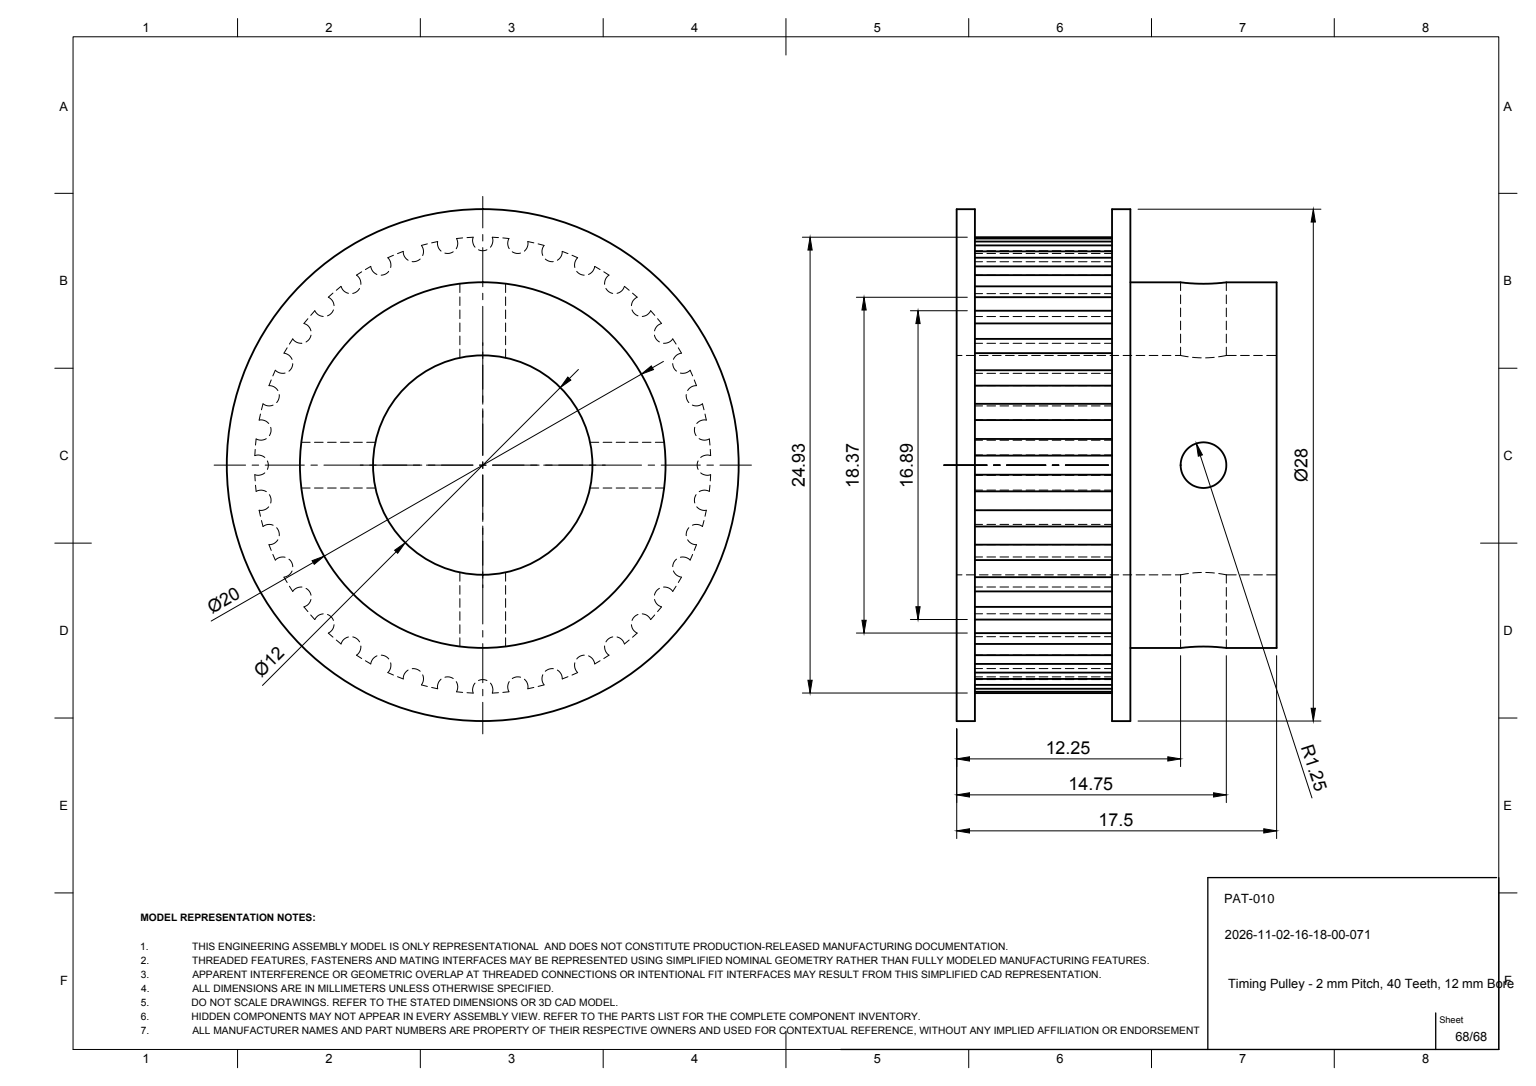
ISO-10303-21;
HEADER;
/* Generated by software containing ST-Developer
 * from STEP Tools, Inc. (www.steptools.com) 
 */

FILE_DESCRIPTION(
/* description */ ('Belt conveyor head drive unit'),
/* implementation_level */ '2;1');

FILE_NAME(
/* name */ 'Timing Pulley - 2 mm Pitch, 40 Teeth, 12 mm Bore.step',
/* time_stamp */ '2026-10-28T03:26:19-07:00',
/* author */ (''),
/* organization */ (''),
/* preprocessor_version */ 'ST-DEVELOPER v20.2',
/* originating_system */ 'Autodesk Translation Framework v15.17.0.0',
/* authorisation */ '');

FILE_SCHEMA (('AUTOMOTIVE_DESIGN { 1 0 10303 214 3 1 1 }'));
ENDSEC;

DATA;
#10=MECHANICAL_DESIGN_GEOMETRIC_PRESENTATION_REPRESENTATION('',(#929),#27069);
#623=B_SPLINE_CURVE_WITH_KNOTS('',3,(#25841,#25842,#25843,#25844,#25845,
#25846,#25847,#25848,#25849,#25850),.UNSPECIFIED.,.F.,.F.,(4,2,2,2,4),(0.565665723963061,
0.61280433739166,0.659942950820258,0.70708195805217,0.754220965284082),
 .UNSPECIFIED.);
#624=B_SPLINE_CURVE_WITH_KNOTS('',3,(#25852,#25853,#25854,#25855,#25856,
#25857,#25858,#25859,#25860,#25861,#25862,#25863,#25864,#25865,#25866,#25867,
#25868,#25869),.UNSPECIFIED.,.F.,.F.,(4,2,2,2,2,2,2,2,4),(0.18855524132102,
0.235693854749619,0.282832468178217,0.329971475410129,0.377110482642041,
0.424249489873953,0.471388497105864,0.518527110534463,0.565665723963061),
 .UNSPECIFIED.);
#625=B_SPLINE_CURVE_WITH_KNOTS('',3,(#25870,#25871,#25872,#25873,#25874,
#25875,#25876,#25877,#25878,#25879),.UNSPECIFIED.,.F.,.F.,(4,2,2,2,4),(0.754220965284082,
0.801359972515993,0.848498979747905,0.895637593176504,0.942776206605102),
 .UNSPECIFIED.);
#626=B_SPLINE_CURVE_WITH_KNOTS('',3,(#25883,#25884,#25885,#25886,#25887,
#25888,#25889,#25890,#25891,#25892),.UNSPECIFIED.,.F.,.F.,(4,2,2,2,4),(0.188940047579712,
0.236173496177583,0.283406944775455,0.330643519967439,0.377880095159423),
 .UNSPECIFIED.);
#627=B_SPLINE_CURVE_WITH_KNOTS('',3,(#25894,#25895,#25896,#25897,#25898,
#25899,#25900,#25901,#25902,#25903),.UNSPECIFIED.,.F.,.F.,(4,2,2,2,4),(0.,
0.0472365751919841,0.0944731503839682,0.14170659898184,0.188940047579712),
 .UNSPECIFIED.);
#628=B_SPLINE_CURVE_WITH_KNOTS('',3,(#25905,#25906,#25907,#25908,#25909,
#25910,#25911,#25912,#25913,#25914),.UNSPECIFIED.,.F.,.F.,(4,2,2,2,4),(0.566820142739135,
0.614053591337007,0.661287039934879,0.708523615126863,0.755760190318847),
 .UNSPECIFIED.);
#629=B_SPLINE_CURVE_WITH_KNOTS('',3,(#25915,#25916,#25917,#25918,#25919,
#25920,#25921,#25922,#25923,#25924),.UNSPECIFIED.,.F.,.F.,(4,2,2,2,4),(0.377880095159423,
0.425116670351408,0.472353245543392,0.519586694141263,0.566820142739135),
 .UNSPECIFIED.);
#630=B_SPLINE_CURVE_WITH_KNOTS('',3,(#25928,#25929,#25930,#25931,#25932,
#25933,#25934,#25935,#25936,#25937,#25938,#25939,#25940,#25941,#25942,#25943,
#25944,#25945),.UNSPECIFIED.,.F.,.F.,(4,2,2,2,2,2,2,2,4),(0.,0.0472365751919841,
0.0944731503839683,0.14170659898184,0.188940047579712,0.236173496177583,
0.283406944775455,0.330643519967439,0.377880095159423),.UNSPECIFIED.);
#631=B_SPLINE_CURVE_WITH_KNOTS('',3,(#25946,#25947,#25948,#25949,#25950,
#25951,#25952,#25953,#25954,#25955,#25956,#25957,#25958,#25959,#25960,#25961,
#25962,#25963),.UNSPECIFIED.,.F.,.F.,(4,2,2,2,2,2,2,2,4),(0.377880095159423,
0.425116670351408,0.472353245543392,0.519586694141263,0.566820142739135,
0.614053591337007,0.661287039934879,0.708523615126863,0.755760190318847),
 .UNSPECIFIED.);
#632=B_SPLINE_CURVE_WITH_KNOTS('',3,(#25967,#25968,#25969,#25970,#25971,
#25972,#25973,#25974,#25975,#25976),.UNSPECIFIED.,.F.,.F.,(4,2,2,2,4),(0.565665723963061,
0.61280433739166,0.659942950820258,0.70708195805217,0.754220965284082),
 .UNSPECIFIED.);
#633=B_SPLINE_CURVE_WITH_KNOTS('',3,(#25978,#25979,#25980,#25981,#25982,
#25983,#25984,#25985,#25986,#25987,#25988,#25989,#25990,#25991,#25992,#25993,
#25994,#25995),.UNSPECIFIED.,.F.,.F.,(4,2,2,2,2,2,2,2,4),(0.18855524132102,
0.235693854749619,0.282832468178217,0.329971475410129,0.377110482642041,
0.424249489873953,0.471388497105864,0.518527110534463,0.565665723963061),
 .UNSPECIFIED.);
#634=B_SPLINE_CURVE_WITH_KNOTS('',3,(#25996,#25997,#25998,#25999,#26000,
#26001,#26002,#26003,#26004,#26005),.UNSPECIFIED.,.F.,.F.,(4,2,2,2,4),(0.754220965284082,
0.801359972515993,0.848498979747905,0.895637593176504,0.942776206605102),
 .UNSPECIFIED.);
#635=B_SPLINE_CURVE_WITH_KNOTS('',3,(#26015,#26016,#26017,#26018,#26019,
#26020,#26021,#26022,#26023,#26024,#26025,#26026,#26027,#26028,#26029,#26030,
#26031,#26032),.UNSPECIFIED.,.F.,.F.,(4,2,2,2,2,2,2,2,4),(0.18855524132102,
0.235693854749619,0.282832468178217,0.329971475410129,0.377110482642041,
0.424249489873953,0.471388497105864,0.518527110534463,0.565665723963061),
 .UNSPECIFIED.);
#636=B_SPLINE_CURVE_WITH_KNOTS('',3,(#26034,#26035,#26036,#26037,#26038,
#26039,#26040,#26041,#26042,#26043),.UNSPECIFIED.,.F.,.F.,(4,2,2,2,4),(0.565665723963061,
0.61280433739166,0.659942950820258,0.70708195805217,0.754220965284082),
 .UNSPECIFIED.);
#637=B_SPLINE_CURVE_WITH_KNOTS('',3,(#26044,#26045,#26046,#26047,#26048,
#26049,#26050,#26051,#26052,#26053),.UNSPECIFIED.,.F.,.F.,(4,2,2,2,4),(0.754220965284082,
0.801359972515993,0.848498979747905,0.895637593176504,0.942776206605102),
 .UNSPECIFIED.);
#638=B_SPLINE_CURVE_WITH_KNOTS('',3,(#26056,#26057,#26058,#26059,#26060,
#26061,#26062,#26063,#26064,#26065,#26066,#26067,#26068,#26069,#26070,#26071,
#26072,#26073),.UNSPECIFIED.,.F.,.F.,(4,2,2,2,2,2,2,2,4),(0.18855524132102,
0.235693854749619,0.282832468178217,0.329971475410129,0.377110482642041,
0.424249489873953,0.471388497105864,0.518527110534463,0.565665723963061),
 .UNSPECIFIED.);
#639=B_SPLINE_CURVE_WITH_KNOTS('',3,(#26075,#26076,#26077,#26078,#26079,
#26080,#26081,#26082,#26083,#26084),.UNSPECIFIED.,.F.,.F.,(4,2,2,2,4),(0.565665723963061,
0.61280433739166,0.659942950820258,0.70708195805217,0.754220965284082),
 .UNSPECIFIED.);
#640=B_SPLINE_CURVE_WITH_KNOTS('',3,(#26085,#26086,#26087,#26088,#26089,
#26090,#26091,#26092,#26093,#26094),.UNSPECIFIED.,.F.,.F.,(4,2,2,2,4),(0.754220965284082,
0.801359972515993,0.848498979747905,0.895637593176504,0.942776206605102),
 .UNSPECIFIED.);
#641=B_SPLINE_CURVE_WITH_KNOTS('',3,(#26099,#26100,#26101,#26102,#26103,
#26104,#26105,#26106,#26107,#26108,#26109,#26110,#26111,#26112,#26113,#26114,
#26115,#26116),.UNSPECIFIED.,.F.,.F.,(4,2,2,2,2,2,2,2,4),(0.,0.0472365751919841,
0.0944731503839683,0.14170659898184,0.188940047579712,0.236173496177583,
0.283406944775455,0.330643519967439,0.377880095159424),.UNSPECIFIED.);
#642=B_SPLINE_CURVE_WITH_KNOTS('',3,(#26117,#26118,#26119,#26120,#26121,
#26122,#26123,#26124,#26125,#26126,#26127,#26128,#26129,#26130,#26131,#26132,
#26133,#26134),.UNSPECIFIED.,.F.,.F.,(4,2,2,2,2,2,2,2,4),(0.377880095159424,
0.425116670351408,0.472353245543392,0.519586694141263,0.566820142739135,
0.614053591337007,0.661287039934879,0.708523615126863,0.755760190318847),
 .UNSPECIFIED.);
#643=B_SPLINE_CURVE_WITH_KNOTS('',3,(#26138,#26139,#26140,#26141,#26142,
#26143,#26144,#26145,#26146,#26147,#26148,#26149,#26150,#26151,#26152,#26153,
#26154,#26155),.UNSPECIFIED.,.F.,.F.,(4,2,2,2,2,2,2,2,4),(0.,0.0472365751919841,
0.0944731503839683,0.14170659898184,0.188940047579712,0.236173496177583,
0.283406944775455,0.330643519967439,0.377880095159423),.UNSPECIFIED.);
#644=B_SPLINE_CURVE_WITH_KNOTS('',3,(#26156,#26157,#26158,#26159,#26160,
#26161,#26162,#26163,#26164,#26165,#26166,#26167,#26168,#26169,#26170,#26171,
#26172,#26173),.UNSPECIFIED.,.F.,.F.,(4,2,2,2,2,2,2,2,4),(0.377880095159423,
0.425116670351408,0.472353245543392,0.519586694141263,0.566820142739135,
0.614053591337007,0.661287039934879,0.708523615126863,0.755760190318847),
 .UNSPECIFIED.);
#775=SHAPE_REPRESENTATION_RELATIONSHIP('SRR','None',#27424,#844);
#844=ADVANCED_BREP_SHAPE_REPRESENTATION('',(#1010),#27066);
#929=STYLED_ITEM('',(#27790),#1010);
#1010=MANIFOLD_SOLID_BREP('Body1',#13798);
#1264=FACE_BOUND('',#3366,.T.);
#1265=FACE_BOUND('',#3367,.T.);
#1266=FACE_BOUND('',#3368,.T.);
#1267=FACE_BOUND('',#3372,.T.);
#1268=FACE_BOUND('',#3373,.T.);
#1269=FACE_BOUND('',#3374,.T.);
#1270=FACE_BOUND('',#3376,.T.);
#1271=FACE_BOUND('',#3378,.T.);
#1272=FACE_BOUND('',#3381,.T.);
#1273=FACE_BOUND('',#3383,.T.);
#1274=FACE_BOUND('',#3386,.T.);
#1608=PLANE('',#16027);
#1609=PLANE('',#16028);
#1610=PLANE('',#16112);
#1611=PLANE('',#16113);
#1612=PLANE('',#16197);
#2311=FACE_OUTER_BOUND('',#3363,.T.);
#2312=FACE_OUTER_BOUND('',#3364,.T.);
#2313=FACE_OUTER_BOUND('',#3365,.T.);
#2314=FACE_OUTER_BOUND('',#3369,.T.);
#2315=FACE_OUTER_BOUND('',#3370,.T.);
#2316=FACE_OUTER_BOUND('',#3371,.T.);
#2317=FACE_OUTER_BOUND('',#3375,.T.);
#2318=FACE_OUTER_BOUND('',#3377,.T.);
#2319=FACE_OUTER_BOUND('',#3379,.T.);
#2320=FACE_OUTER_BOUND('',#3380,.T.);
#2321=FACE_OUTER_BOUND('',#3382,.T.);
#2322=FACE_OUTER_BOUND('',#3384,.T.);
#2323=FACE_OUTER_BOUND('',#3385,.T.);
#2324=FACE_OUTER_BOUND('',#3387,.T.);
#2325=FACE_OUTER_BOUND('',#3388,.T.);
#2326=FACE_OUTER_BOUND('',#3389,.T.);
#2327=FACE_OUTER_BOUND('',#3390,.T.);
#2328=FACE_OUTER_BOUND('',#3391,.T.);
#2329=FACE_OUTER_BOUND('',#3392,.T.);
#2330=FACE_OUTER_BOUND('',#3393,.T.);
#2331=FACE_OUTER_BOUND('',#3394,.T.);
#2332=FACE_OUTER_BOUND('',#3395,.T.);
#2333=FACE_OUTER_BOUND('',#3396,.T.);
#2334=FACE_OUTER_BOUND('',#3397,.T.);
#2335=FACE_OUTER_BOUND('',#3398,.T.);
#2336=FACE_OUTER_BOUND('',#3399,.T.);
#2337=FACE_OUTER_BOUND('',#3400,.T.);
#2338=FACE_OUTER_BOUND('',#3401,.T.);
#2339=FACE_OUTER_BOUND('',#3402,.T.);
#2340=FACE_OUTER_BOUND('',#3403,.T.);
#2341=FACE_OUTER_BOUND('',#3404,.T.);
#2342=FACE_OUTER_BOUND('',#3405,.T.);
#2343=FACE_OUTER_BOUND('',#3406,.T.);
#2344=FACE_OUTER_BOUND('',#3407,.T.);
#2345=FACE_OUTER_BOUND('',#3408,.T.);
#2346=FACE_OUTER_BOUND('',#3409,.T.);
#2347=FACE_OUTER_BOUND('',#3410,.T.);
#2348=FACE_OUTER_BOUND('',#3411,.T.);
#2349=FACE_OUTER_BOUND('',#3412,.T.);
#2350=FACE_OUTER_BOUND('',#3413,.T.);
#2351=FACE_OUTER_BOUND('',#3414,.T.);
#2352=FACE_OUTER_BOUND('',#3415,.T.);
#2353=FACE_OUTER_BOUND('',#3416,.T.);
#2354=FACE_OUTER_BOUND('',#3417,.T.);
#2355=FACE_OUTER_BOUND('',#3418,.T.);
#2356=FACE_OUTER_BOUND('',#3419,.T.);
#2357=FACE_OUTER_BOUND('',#3420,.T.);
#2358=FACE_OUTER_BOUND('',#3421,.T.);
#2359=FACE_OUTER_BOUND('',#3422,.T.);
#2360=FACE_OUTER_BOUND('',#3423,.T.);
#2361=FACE_OUTER_BOUND('',#3424,.T.);
#2362=FACE_OUTER_BOUND('',#3425,.T.);
#2363=FACE_OUTER_BOUND('',#3426,.T.);
#2364=FACE_OUTER_BOUND('',#3427,.T.);
#2365=FACE_OUTER_BOUND('',#3428,.T.);
#2366=FACE_OUTER_BOUND('',#3429,.T.);
#2367=FACE_OUTER_BOUND('',#3430,.T.);
#2368=FACE_OUTER_BOUND('',#3431,.T.);
#2369=FACE_OUTER_BOUND('',#3432,.T.);
#2370=FACE_OUTER_BOUND('',#3433,.T.);
#2371=FACE_OUTER_BOUND('',#3434,.T.);
#2372=FACE_OUTER_BOUND('',#3435,.T.);
#2373=FACE_OUTER_BOUND('',#3436,.T.);
#2374=FACE_OUTER_BOUND('',#3437,.T.);
#2375=FACE_OUTER_BOUND('',#3438,.T.);
#2376=FACE_OUTER_BOUND('',#3439,.T.);
#2377=FACE_OUTER_BOUND('',#3440,.T.);
#2378=FACE_OUTER_BOUND('',#3441,.T.);
#2379=FACE_OUTER_BOUND('',#3442,.T.);
#2380=FACE_OUTER_BOUND('',#3443,.T.);
#2381=FACE_OUTER_BOUND('',#3444,.T.);
#2382=FACE_OUTER_BOUND('',#3445,.T.);
#2383=FACE_OUTER_BOUND('',#3446,.T.);
#2384=FACE_OUTER_BOUND('',#3447,.T.);
#2385=FACE_OUTER_BOUND('',#3448,.T.);
#2386=FACE_OUTER_BOUND('',#3449,.T.);
#2387=FACE_OUTER_BOUND('',#3450,.T.);
#2388=FACE_OUTER_BOUND('',#3451,.T.);
#2389=FACE_OUTER_BOUND('',#3452,.T.);
#2390=FACE_OUTER_BOUND('',#3453,.T.);
#2391=FACE_OUTER_BOUND('',#3454,.T.);
#2392=FACE_OUTER_BOUND('',#3455,.T.);
#2393=FACE_OUTER_BOUND('',#3456,.T.);
#2394=FACE_OUTER_BOUND('',#3457,.T.);
#2395=FACE_OUTER_BOUND('',#3458,.T.);
#2396=FACE_OUTER_BOUND('',#3459,.T.);
#2397=FACE_OUTER_BOUND('',#3460,.T.);
#2398=FACE_OUTER_BOUND('',#3461,.T.);
#2399=FACE_OUTER_BOUND('',#3462,.T.);
#2400=FACE_OUTER_BOUND('',#3463,.T.);
#2401=FACE_OUTER_BOUND('',#3464,.T.);
#2402=FACE_OUTER_BOUND('',#3465,.T.);
#2403=FACE_OUTER_BOUND('',#3466,.T.);
#3363=EDGE_LOOP('',(#11858,#11859,#11860,#11861,#11862,#11863,#11864,#11865,
#11866));
#3364=EDGE_LOOP('',(#11867,#11868,#11869,#11870,#11871,#11872,#11873));
#3365=EDGE_LOOP('',(#11874,#11875,#11876,#11877,#11878,#11879,#11880,#11881,
#11882));
#3366=EDGE_LOOP('',(#11883,#11884,#11885));
#3367=EDGE_LOOP('',(#11886,#11887,#11888));
#3368=EDGE_LOOP('',(#11889,#11890,#11891));
#3369=EDGE_LOOP('',(#11892,#11893,#11894,#11895,#11896,#11897,#11898));
#3370=EDGE_LOOP('',(#11899,#11900,#11901,#11902,#11903,#11904,#11905));
#3371=EDGE_LOOP('',(#11906,#11907,#11908,#11909,#11910,#11911,#11912,#11913,
#11914,#11915));
#3372=EDGE_LOOP('',(#11916,#11917));
#3373=EDGE_LOOP('',(#11918,#11919));
#3374=EDGE_LOOP('',(#11920,#11921));
#3375=EDGE_LOOP('',(#11922));
#3376=EDGE_LOOP('',(#11923));
#3377=EDGE_LOOP('',(#11924));
#3378=EDGE_LOOP('',(#11925,#11926,#11927,#11928,#11929,#11930,#11931,#11932,
#11933,#11934,#11935,#11936,#11937,#11938,#11939,#11940,#11941,#11942,#11943,
#11944,#11945,#11946,#11947,#11948,#11949,#11950,#11951,#11952,#11953,#11954,
#11955,#11956,#11957,#11958,#11959,#11960,#11961,#11962,#11963,#11964,#11965,
#11966,#11967,#11968,#11969,#11970,#11971,#11972,#11973,#11974,#11975,#11976,
#11977,#11978,#11979,#11980,#11981,#11982,#11983,#11984,#11985,#11986,#11987,
#11988,#11989,#11990,#11991,#11992,#11993,#11994,#11995,#11996,#11997,#11998,
#11999,#12000,#12001,#12002,#12003,#12004));
#3379=EDGE_LOOP('',(#12005,#12006,#12007,#12008));
#3380=EDGE_LOOP('',(#12009));
#3381=EDGE_LOOP('',(#12010));
#3382=EDGE_LOOP('',(#12011));
#3383=EDGE_LOOP('',(#12012,#12013,#12014,#12015,#12016,#12017,#12018,#12019,
#12020,#12021,#12022,#12023,#12024,#12025,#12026,#12027,#12028,#12029,#12030,
#12031,#12032,#12033,#12034,#12035,#12036,#12037,#12038,#12039,#12040,#12041,
#12042,#12043,#12044,#12045,#12046,#12047,#12048,#12049,#12050,#12051,#12052,
#12053,#12054,#12055,#12056,#12057,#12058,#12059,#12060,#12061,#12062,#12063,
#12064,#12065,#12066,#12067,#12068,#12069,#12070,#12071,#12072,#12073,#12074,
#12075,#12076,#12077,#12078,#12079,#12080,#12081,#12082,#12083,#12084,#12085,
#12086,#12087,#12088,#12089,#12090,#12091));
#3384=EDGE_LOOP('',(#12092,#12093,#12094,#12095));
#3385=EDGE_LOOP('',(#12096));
#3386=EDGE_LOOP('',(#12097));
#3387=EDGE_LOOP('',(#12098,#12099,#12100,#12101));
#3388=EDGE_LOOP('',(#12102,#12103,#12104,#12105));
#3389=EDGE_LOOP('',(#12106,#12107,#12108,#12109));
#3390=EDGE_LOOP('',(#12110,#12111,#12112,#12113));
#3391=EDGE_LOOP('',(#12114,#12115,#12116,#12117));
#3392=EDGE_LOOP('',(#12118,#12119,#12120,#12121));
#3393=EDGE_LOOP('',(#12122,#12123,#12124,#12125));
#3394=EDGE_LOOP('',(#12126,#12127,#12128,#12129));
#3395=EDGE_LOOP('',(#12130,#12131,#12132,#12133));
#3396=EDGE_LOOP('',(#12134,#12135,#12136,#12137));
#3397=EDGE_LOOP('',(#12138,#12139,#12140,#12141));
#3398=EDGE_LOOP('',(#12142,#12143,#12144,#12145));
#3399=EDGE_LOOP('',(#12146,#12147,#12148,#12149));
#3400=EDGE_LOOP('',(#12150,#12151,#12152,#12153));
#3401=EDGE_LOOP('',(#12154,#12155,#12156,#12157));
#3402=EDGE_LOOP('',(#12158,#12159,#12160,#12161));
#3403=EDGE_LOOP('',(#12162,#12163,#12164,#12165));
#3404=EDGE_LOOP('',(#12166,#12167,#12168,#12169));
#3405=EDGE_LOOP('',(#12170,#12171,#12172,#12173));
#3406=EDGE_LOOP('',(#12174,#12175,#12176,#12177));
#3407=EDGE_LOOP('',(#12178,#12179,#12180,#12181));
#3408=EDGE_LOOP('',(#12182,#12183,#12184,#12185));
#3409=EDGE_LOOP('',(#12186,#12187,#12188,#12189));
#3410=EDGE_LOOP('',(#12190,#12191,#12192,#12193));
#3411=EDGE_LOOP('',(#12194,#12195,#12196,#12197));
#3412=EDGE_LOOP('',(#12198,#12199,#12200,#12201));
#3413=EDGE_LOOP('',(#12202,#12203,#12204,#12205));
#3414=EDGE_LOOP('',(#12206,#12207,#12208,#12209));
#3415=EDGE_LOOP('',(#12210,#12211,#12212,#12213));
#3416=EDGE_LOOP('',(#12214,#12215,#12216,#12217));
#3417=EDGE_LOOP('',(#12218,#12219,#12220,#12221));
#3418=EDGE_LOOP('',(#12222,#12223,#12224,#12225));
#3419=EDGE_LOOP('',(#12226,#12227,#12228,#12229));
#3420=EDGE_LOOP('',(#12230,#12231,#12232,#12233));
#3421=EDGE_LOOP('',(#12234,#12235,#12236,#12237));
#3422=EDGE_LOOP('',(#12238,#12239,#12240,#12241));
#3423=EDGE_LOOP('',(#12242,#12243,#12244,#12245));
#3424=EDGE_LOOP('',(#12246,#12247,#12248,#12249));
#3425=EDGE_LOOP('',(#12250,#12251,#12252,#12253));
#3426=EDGE_LOOP('',(#12254,#12255,#12256,#12257));
#3427=EDGE_LOOP('',(#12258,#12259,#12260,#12261));
#3428=EDGE_LOOP('',(#12262,#12263,#12264,#12265));
#3429=EDGE_LOOP('',(#12266,#12267,#12268,#12269));
#3430=EDGE_LOOP('',(#12270,#12271,#12272,#12273));
#3431=EDGE_LOOP('',(#12274,#12275,#12276,#12277));
#3432=EDGE_LOOP('',(#12278,#12279,#12280,#12281));
#3433=EDGE_LOOP('',(#12282,#12283,#12284,#12285));
#3434=EDGE_LOOP('',(#12286,#12287,#12288,#12289));
#3435=EDGE_LOOP('',(#12290,#12291,#12292,#12293));
#3436=EDGE_LOOP('',(#12294,#12295,#12296,#12297));
#3437=EDGE_LOOP('',(#12298,#12299,#12300,#12301));
#3438=EDGE_LOOP('',(#12302,#12303,#12304,#12305));
#3439=EDGE_LOOP('',(#12306,#12307,#12308,#12309));
#3440=EDGE_LOOP('',(#12310,#12311,#12312,#12313));
#3441=EDGE_LOOP('',(#12314,#12315,#12316,#12317));
#3442=EDGE_LOOP('',(#12318,#12319,#12320,#12321));
#3443=EDGE_LOOP('',(#12322,#12323,#12324,#12325));
#3444=EDGE_LOOP('',(#12326,#12327,#12328,#12329));
#3445=EDGE_LOOP('',(#12330,#12331,#12332,#12333));
#3446=EDGE_LOOP('',(#12334,#12335,#12336,#12337));
#3447=EDGE_LOOP('',(#12338,#12339,#12340,#12341));
#3448=EDGE_LOOP('',(#12342,#12343,#12344,#12345));
#3449=EDGE_LOOP('',(#12346,#12347,#12348,#12349));
#3450=EDGE_LOOP('',(#12350,#12351,#12352,#12353));
#3451=EDGE_LOOP('',(#12354,#12355,#12356,#12357));
#3452=EDGE_LOOP('',(#12358,#12359,#12360,#12361));
#3453=EDGE_LOOP('',(#12362,#12363,#12364,#12365));
#3454=EDGE_LOOP('',(#12366,#12367,#12368,#12369));
#3455=EDGE_LOOP('',(#12370,#12371,#12372,#12373));
#3456=EDGE_LOOP('',(#12374,#12375,#12376,#12377));
#3457=EDGE_LOOP('',(#12378,#12379,#12380,#12381));
#3458=EDGE_LOOP('',(#12382,#12383,#12384,#12385));
#3459=EDGE_LOOP('',(#12386,#12387,#12388,#12389));
#3460=EDGE_LOOP('',(#12390,#12391,#12392,#12393));
#3461=EDGE_LOOP('',(#12394,#12395,#12396,#12397));
#3462=EDGE_LOOP('',(#12398,#12399,#12400,#12401));
#3463=EDGE_LOOP('',(#12402,#12403,#12404,#12405));
#3464=EDGE_LOOP('',(#12406,#12407,#12408,#12409));
#3465=EDGE_LOOP('',(#12410,#12411,#12412,#12413));
#3466=EDGE_LOOP('',(#12414,#12415,#12416,#12417));
#4155=LINE('',#25881,#4947);
#4156=LINE('',#25965,#4948);
#4157=LINE('',#26009,#4949);
#4158=LINE('',#26011,#4950);
#4159=LINE('',#26097,#4951);
#4160=LINE('',#26174,#4952);
#4161=LINE('',#26178,#4953);
#4162=LINE('',#26180,#4954);
#4163=LINE('',#26349,#4955);
#4164=LINE('',#26517,#4956);
#4165=LINE('',#26520,#4957);
#4166=LINE('',#26521,#4958);
#4167=LINE('',#26523,#4959);
#4168=LINE('',#26525,#4960);
#4169=LINE('',#26527,#4961);
#4170=LINE('',#26529,#4962);
#4171=LINE('',#26531,#4963);
#4172=LINE('',#26533,#4964);
#4173=LINE('',#26535,#4965);
#4174=LINE('',#26537,#4966);
#4175=LINE('',#26539,#4967);
#4176=LINE('',#26541,#4968);
#4177=LINE('',#26543,#4969);
#4178=LINE('',#26545,#4970);
#4179=LINE('',#26547,#4971);
#4180=LINE('',#26549,#4972);
#4181=LINE('',#26551,#4973);
#4182=LINE('',#26553,#4974);
#4183=LINE('',#26555,#4975);
#4184=LINE('',#26557,#4976);
#4185=LINE('',#26559,#4977);
#4186=LINE('',#26561,#4978);
#4187=LINE('',#26563,#4979);
#4188=LINE('',#26565,#4980);
#4189=LINE('',#26567,#4981);
#4190=LINE('',#26569,#4982);
#4191=LINE('',#26571,#4983);
#4192=LINE('',#26573,#4984);
#4193=LINE('',#26575,#4985);
#4194=LINE('',#26577,#4986);
#4195=LINE('',#26579,#4987);
#4196=LINE('',#26581,#4988);
#4197=LINE('',#26583,#4989);
#4198=LINE('',#26585,#4990);
#4199=LINE('',#26587,#4991);
#4200=LINE('',#26589,#4992);
#4201=LINE('',#26591,#4993);
#4202=LINE('',#26593,#4994);
#4203=LINE('',#26595,#4995);
#4204=LINE('',#26597,#4996);
#4205=LINE('',#26599,#4997);
#4206=LINE('',#26601,#4998);
#4207=LINE('',#26603,#4999);
#4208=LINE('',#26605,#5000);
#4209=LINE('',#26607,#5001);
#4210=LINE('',#26609,#5002);
#4211=LINE('',#26611,#5003);
#4212=LINE('',#26613,#5004);
#4213=LINE('',#26615,#5005);
#4214=LINE('',#26617,#5006);
#4215=LINE('',#26619,#5007);
#4216=LINE('',#26621,#5008);
#4217=LINE('',#26623,#5009);
#4218=LINE('',#26625,#5010);
#4219=LINE('',#26627,#5011);
#4220=LINE('',#26629,#5012);
#4221=LINE('',#26631,#5013);
#4222=LINE('',#26633,#5014);
#4223=LINE('',#26635,#5015);
#4224=LINE('',#26637,#5016);
#4225=LINE('',#26639,#5017);
#4226=LINE('',#26641,#5018);
#4227=LINE('',#26643,#5019);
#4228=LINE('',#26645,#5020);
#4229=LINE('',#26647,#5021);
#4230=LINE('',#26649,#5022);
#4231=LINE('',#26651,#5023);
#4232=LINE('',#26653,#5024);
#4233=LINE('',#26655,#5025);
#4234=LINE('',#26657,#5026);
#4235=LINE('',#26659,#5027);
#4236=LINE('',#26661,#5028);
#4237=LINE('',#26663,#5029);
#4238=LINE('',#26665,#5030);
#4239=LINE('',#26667,#5031);
#4240=LINE('',#26669,#5032);
#4241=LINE('',#26671,#5033);
#4242=LINE('',#26673,#5034);
#4243=LINE('',#26675,#5035);
#4244=LINE('',#26677,#5036);
#4947=VECTOR('',#20003,0.125);
#4948=VECTOR('',#20006,0.125);
#4949=VECTOR('',#20011,1.);
#4950=VECTOR('',#20012,1.);
#4951=VECTOR('',#20017,0.125);
#4952=VECTOR('',#20020,0.125);
#4953=VECTOR('',#20025,0.6);
#4954=VECTOR('',#20026,0.6);
#4955=VECTOR('',#20199,1.4);
#4956=VECTOR('',#20370,1.4);
#4957=VECTOR('',#20375,1.);
#4958=VECTOR('',#20376,1.);
#4959=VECTOR('',#20379,1.);
#4960=VECTOR('',#20382,1.);
#4961=VECTOR('',#20385,1.);
#4962=VECTOR('',#20388,1.);
#4963=VECTOR('',#20391,1.);
#4964=VECTOR('',#20394,1.);
#4965=VECTOR('',#20397,1.);
#4966=VECTOR('',#20400,1.);
#4967=VECTOR('',#20403,1.);
#4968=VECTOR('',#20406,1.);
#4969=VECTOR('',#20409,1.);
#4970=VECTOR('',#20412,1.);
#4971=VECTOR('',#20415,1.);
#4972=VECTOR('',#20418,1.);
#4973=VECTOR('',#20421,1.);
#4974=VECTOR('',#20424,1.);
#4975=VECTOR('',#20427,1.);
#4976=VECTOR('',#20430,1.);
#4977=VECTOR('',#20433,1.);
#4978=VECTOR('',#20436,1.);
#4979=VECTOR('',#20439,1.);
#4980=VECTOR('',#20442,1.);
#4981=VECTOR('',#20445,1.);
#4982=VECTOR('',#20448,1.);
#4983=VECTOR('',#20451,1.);
#4984=VECTOR('',#20454,1.);
#4985=VECTOR('',#20457,1.);
#4986=VECTOR('',#20460,1.);
#4987=VECTOR('',#20463,1.);
#4988=VECTOR('',#20466,1.);
#4989=VECTOR('',#20469,1.);
#4990=VECTOR('',#20472,1.);
#4991=VECTOR('',#20475,1.);
#4992=VECTOR('',#20478,1.);
#4993=VECTOR('',#20481,1.);
#4994=VECTOR('',#20484,1.);
#4995=VECTOR('',#20487,1.);
#4996=VECTOR('',#20490,1.);
#4997=VECTOR('',#20493,1.);
#4998=VECTOR('',#20496,1.);
#4999=VECTOR('',#20499,1.);
#5000=VECTOR('',#20502,1.);
#5001=VECTOR('',#20505,1.);
#5002=VECTOR('',#20508,1.);
#5003=VECTOR('',#20511,1.);
#5004=VECTOR('',#20514,1.);
#5005=VECTOR('',#20517,1.);
#5006=VECTOR('',#20520,1.);
#5007=VECTOR('',#20523,1.);
#5008=VECTOR('',#20526,1.);
#5009=VECTOR('',#20529,1.);
#5010=VECTOR('',#20532,1.);
#5011=VECTOR('',#20535,1.);
#5012=VECTOR('',#20538,1.);
#5013=VECTOR('',#20541,1.);
#5014=VECTOR('',#20544,1.);
#5015=VECTOR('',#20547,1.);
#5016=VECTOR('',#20550,1.);
#5017=VECTOR('',#20553,1.);
#5018=VECTOR('',#20556,1.);
#5019=VECTOR('',#20559,1.);
#5020=VECTOR('',#20562,1.);
#5021=VECTOR('',#20565,1.);
#5022=VECTOR('',#20568,1.);
#5023=VECTOR('',#20571,1.);
#5024=VECTOR('',#20574,1.);
#5025=VECTOR('',#20577,1.);
#5026=VECTOR('',#20580,1.);
#5027=VECTOR('',#20583,1.);
#5028=VECTOR('',#20586,1.);
#5029=VECTOR('',#20589,1.);
#5030=VECTOR('',#20592,1.);
#5031=VECTOR('',#20595,1.);
#5032=VECTOR('',#20598,1.);
#5033=VECTOR('',#20601,1.);
#5034=VECTOR('',#20604,1.);
#5035=VECTOR('',#20607,1.);
#5036=VECTOR('',#20610,1.);
#5773=CIRCLE('',#16020,1.);
#5774=CIRCLE('',#16021,1.);
#5775=CIRCLE('',#16025,0.6);
#5776=CIRCLE('',#16026,0.6);
#5777=CIRCLE('',#16029,1.4);
#5778=CIRCLE('',#16030,0.0555000000000001);
#5779=CIRCLE('',#16031,1.24783954473516);
#5780=CIRCLE('',#16032,0.0555000000000001);
#5781=CIRCLE('',#16033,1.24783954473516);
#5782=CIRCLE('',#16034,0.0555000000000001);
#5783=CIRCLE('',#16035,1.24783954473516);
#5784=CIRCLE('',#16036,0.0555000000000001);
#5785=CIRCLE('',#16037,1.24783954473516);
#5786=CIRCLE('',#16038,0.0555000000000001);
#5787=CIRCLE('',#16039,1.24783954473516);
#5788=CIRCLE('',#16040,0.0555000000000001);
#5789=CIRCLE('',#16041,1.24783954473516);
#5790=CIRCLE('',#16042,0.0555000000000001);
#5791=CIRCLE('',#16043,1.24783954473516);
#5792=CIRCLE('',#16044,0.0555000000000001);
#5793=CIRCLE('',#16045,1.24783954473516);
#5794=CIRCLE('',#16046,0.0555000000000001);
#5795=CIRCLE('',#16047,1.24783954473516);
#5796=CIRCLE('',#16048,0.0555000000000001);
#5797=CIRCLE('',#16049,1.24783954473516);
#5798=CIRCLE('',#16050,0.0555000000000001);
#5799=CIRCLE('',#16051,1.24783954473516);
#5800=CIRCLE('',#16052,0.0555000000000001);
#5801=CIRCLE('',#16053,1.24783954473516);
#5802=CIRCLE('',#16054,0.0555000000000001);
#5803=CIRCLE('',#16055,1.24783954473516);
#5804=CIRCLE('',#16056,0.0555000000000001);
#5805=CIRCLE('',#16057,1.24783954473516);
#5806=CIRCLE('',#16058,0.0555000000000001);
#5807=CIRCLE('',#16059,1.24783954473516);
#5808=CIRCLE('',#16060,0.0555000000000001);
#5809=CIRCLE('',#16061,1.24783954473516);
#5810=CIRCLE('',#16062,0.0555000000000001);
#5811=CIRCLE('',#16063,1.24783954473516);
#5812=CIRCLE('',#16064,0.0555000000000001);
#5813=CIRCLE('',#16065,1.24783954473516);
#5814=CIRCLE('',#16066,0.0555000000000001);
#5815=CIRCLE('',#16067,1.24783954473516);
#5816=CIRCLE('',#16068,0.0555000000000001);
#5817=CIRCLE('',#16069,1.24783954473516);
#5818=CIRCLE('',#16070,0.0555000000000001);
#5819=CIRCLE('',#16071,1.24783954473516);
#5820=CIRCLE('',#16072,0.0555000000000001);
#5821=CIRCLE('',#16073,1.24783954473516);
#5822=CIRCLE('',#16074,0.0555000000000001);
#5823=CIRCLE('',#16075,1.24783954473516);
#5824=CIRCLE('',#16076,0.0555000000000001);
#5825=CIRCLE('',#16077,1.24783954473516);
#5826=CIRCLE('',#16078,0.0555000000000001);
#5827=CIRCLE('',#16079,1.24783954473516);
#5828=CIRCLE('',#16080,0.0555000000000001);
#5829=CIRCLE('',#16081,1.24783954473516);
#5830=CIRCLE('',#16082,0.0555000000000001);
#5831=CIRCLE('',#16083,1.24783954473516);
#5832=CIRCLE('',#16084,0.0555000000000001);
#5833=CIRCLE('',#16085,1.24783954473516);
#5834=CIRCLE('',#16086,0.0555000000000001);
#5835=CIRCLE('',#16087,1.24783954473516);
#5836=CIRCLE('',#16088,0.0555000000000001);
#5837=CIRCLE('',#16089,1.24783954473516);
#5838=CIRCLE('',#16090,0.0555000000000001);
#5839=CIRCLE('',#16091,1.24783954473516);
#5840=CIRCLE('',#16092,0.0555000000000001);
#5841=CIRCLE('',#16093,1.24783954473516);
#5842=CIRCLE('',#16094,0.0555000000000001);
#5843=CIRCLE('',#16095,1.24783954473516);
#5844=CIRCLE('',#16096,0.0555000000000001);
#5845=CIRCLE('',#16097,1.24783954473516);
#5846=CIRCLE('',#16098,0.0555000000000001);
#5847=CIRCLE('',#16099,1.24783954473516);
#5848=CIRCLE('',#16100,0.0555000000000001);
#5849=CIRCLE('',#16101,1.24783954473516);
#5850=CIRCLE('',#16102,0.0555000000000001);
#5851=CIRCLE('',#16103,1.24783954473516);
#5852=CIRCLE('',#16104,0.0555000000000001);
#5853=CIRCLE('',#16105,1.24783954473516);
#5854=CIRCLE('',#16106,0.0555000000000001);
#5855=CIRCLE('',#16107,1.24783954473516);
#5856=CIRCLE('',#16108,0.0555000000000001);
#5857=CIRCLE('',#16109,1.24783954473516);
#5858=CIRCLE('',#16111,1.4);
#5859=CIRCLE('',#16114,1.4);
#5860=CIRCLE('',#16115,0.0555000000000001);
#5861=CIRCLE('',#16116,1.24783954473516);
#5862=CIRCLE('',#16117,0.0555000000000001);
#5863=CIRCLE('',#16118,1.24783954473516);
#5864=CIRCLE('',#16119,0.0555000000000001);
#5865=CIRCLE('',#16120,1.24783954473516);
#5866=CIRCLE('',#16121,0.0555000000000001);
#5867=CIRCLE('',#16122,1.24783954473516);
#5868=CIRCLE('',#16123,0.0555000000000001);
#5869=CIRCLE('',#16124,1.24783954473516);
#5870=CIRCLE('',#16125,0.0555000000000001);
#5871=CIRCLE('',#16126,1.24783954473516);
#5872=CIRCLE('',#16127,0.0555000000000001);
#5873=CIRCLE('',#16128,1.24783954473516);
#5874=CIRCLE('',#16129,0.0555000000000001);
#5875=CIRCLE('',#16130,1.24783954473516);
#5876=CIRCLE('',#16131,0.0555000000000001);
#5877=CIRCLE('',#16132,1.24783954473516);
#5878=CIRCLE('',#16133,0.0555000000000001);
#5879=CIRCLE('',#16134,1.24783954473516);
#5880=CIRCLE('',#16135,0.0555000000000001);
#5881=CIRCLE('',#16136,1.24783954473516);
#5882=CIRCLE('',#16137,0.0555000000000001);
#5883=CIRCLE('',#16138,1.24783954473516);
#5884=CIRCLE('',#16139,0.0555000000000001);
#5885=CIRCLE('',#16140,1.24783954473516);
#5886=CIRCLE('',#16141,0.0555000000000001);
#5887=CIRCLE('',#16142,1.24783954473516);
#5888=CIRCLE('',#16143,0.0555000000000001);
#5889=CIRCLE('',#16144,1.24783954473516);
#5890=CIRCLE('',#16145,0.0555000000000001);
#5891=CIRCLE('',#16146,1.24783954473516);
#5892=CIRCLE('',#16147,0.0555000000000001);
#5893=CIRCLE('',#16148,1.24783954473516);
#5894=CIRCLE('',#16149,0.0555000000000001);
#5895=CIRCLE('',#16150,1.24783954473516);
#5896=CIRCLE('',#16151,0.0555000000000001);
#5897=CIRCLE('',#16152,1.24783954473516);
#5898=CIRCLE('',#16153,0.0555000000000001);
#5899=CIRCLE('',#16154,1.24783954473516);
#5900=CIRCLE('',#16155,0.0555000000000001);
#5901=CIRCLE('',#16156,1.24783954473516);
#5902=CIRCLE('',#16157,0.0555000000000001);
#5903=CIRCLE('',#16158,1.24783954473516);
#5904=CIRCLE('',#16159,0.0555000000000001);
#5905=CIRCLE('',#16160,1.24783954473516);
#5906=CIRCLE('',#16161,0.0555000000000001);
#5907=CIRCLE('',#16162,1.24783954473516);
#5908=CIRCLE('',#16163,0.0555000000000001);
#5909=CIRCLE('',#16164,1.24783954473516);
#5910=CIRCLE('',#16165,0.0555000000000001);
#5911=CIRCLE('',#16166,1.24783954473516);
#5912=CIRCLE('',#16167,0.0555000000000001);
#5913=CIRCLE('',#16168,1.24783954473516);
#5914=CIRCLE('',#16169,0.0555000000000001);
#5915=CIRCLE('',#16170,1.24783954473516);
#5916=CIRCLE('',#16171,0.0555000000000001);
#5917=CIRCLE('',#16172,1.24783954473516);
#5918=CIRCLE('',#16173,0.0555000000000001);
#5919=CIRCLE('',#16174,1.24783954473516);
#5920=CIRCLE('',#16175,0.0555000000000001);
#5921=CIRCLE('',#16176,1.24783954473516);
#5922=CIRCLE('',#16177,0.0555000000000001);
#5923=CIRCLE('',#16178,1.24783954473516);
#5924=CIRCLE('',#16179,0.0555000000000001);
#5925=CIRCLE('',#16180,1.24783954473516);
#5926=CIRCLE('',#16181,0.0555000000000001);
#5927=CIRCLE('',#16182,1.24783954473516);
#5928=CIRCLE('',#16183,0.0555000000000001);
#5929=CIRCLE('',#16184,1.24783954473516);
#5930=CIRCLE('',#16185,0.0555000000000001);
#5931=CIRCLE('',#16186,1.24783954473516);
#5932=CIRCLE('',#16187,0.0555000000000001);
#5933=CIRCLE('',#16188,1.24783954473516);
#5934=CIRCLE('',#16189,0.0555000000000001);
#5935=CIRCLE('',#16190,1.24783954473516);
#5936=CIRCLE('',#16191,0.0555000000000001);
#5937=CIRCLE('',#16192,1.24783954473516);
#5938=CIRCLE('',#16193,0.0555000000000001);
#5939=CIRCLE('',#16194,1.24783954473516);
#5940=CIRCLE('',#16196,1.4);
#6945=VERTEX_POINT('',#25839);
#6946=VERTEX_POINT('',#25840);
#6947=VERTEX_POINT('',#25851);
#6948=VERTEX_POINT('',#25880);
#6949=VERTEX_POINT('',#25882);
#6950=VERTEX_POINT('',#25893);
#6951=VERTEX_POINT('',#25904);
#6952=VERTEX_POINT('',#25926);
#6953=VERTEX_POINT('',#25927);
#6954=VERTEX_POINT('',#25964);
#6955=VERTEX_POINT('',#25966);
#6956=VERTEX_POINT('',#25977);
#6957=VERTEX_POINT('',#26007);
#6958=VERTEX_POINT('',#26010);
#6959=VERTEX_POINT('',#26013);
#6960=VERTEX_POINT('',#26014);
#6961=VERTEX_POINT('',#26033);
#6962=VERTEX_POINT('',#26054);
#6963=VERTEX_POINT('',#26055);
#6964=VERTEX_POINT('',#26074);
#6965=VERTEX_POINT('',#26096);
#6966=VERTEX_POINT('',#26098);
#6967=VERTEX_POINT('',#26136);
#6968=VERTEX_POINT('',#26137);
#6969=VERTEX_POINT('',#26176);
#6970=VERTEX_POINT('',#26179);
#6971=VERTEX_POINT('',#26184);
#6972=VERTEX_POINT('',#26186);
#6973=VERTEX_POINT('',#26187);
#6974=VERTEX_POINT('',#26189);
#6975=VERTEX_POINT('',#26191);
#6976=VERTEX_POINT('',#26193);
#6977=VERTEX_POINT('',#26195);
#6978=VERTEX_POINT('',#26197);
#6979=VERTEX_POINT('',#26199);
#6980=VERTEX_POINT('',#26201);
#6981=VERTEX_POINT('',#26203);
#6982=VERTEX_POINT('',#26205);
#6983=VERTEX_POINT('',#26207);
#6984=VERTEX_POINT('',#26209);
#6985=VERTEX_POINT('',#26211);
#6986=VERTEX_POINT('',#26213);
#6987=VERTEX_POINT('',#26215);
#6988=VERTEX_POINT('',#26217);
#6989=VERTEX_POINT('',#26219);
#6990=VERTEX_POINT('',#26221);
#6991=VERTEX_POINT('',#26223);
#6992=VERTEX_POINT('',#26225);
#6993=VERTEX_POINT('',#26227);
#6994=VERTEX_POINT('',#26229);
#6995=VERTEX_POINT('',#26231);
#6996=VERTEX_POINT('',#26233);
#6997=VERTEX_POINT('',#26235);
#6998=VERTEX_POINT('',#26237);
#6999=VERTEX_POINT('',#26239);
#7000=VERTEX_POINT('',#26241);
#7001=VERTEX_POINT('',#26243);
#7002=VERTEX_POINT('',#26245);
#7003=VERTEX_POINT('',#26247);
#7004=VERTEX_POINT('',#26249);
#7005=VERTEX_POINT('',#26251);
#7006=VERTEX_POINT('',#26253);
#7007=VERTEX_POINT('',#26255);
#7008=VERTEX_POINT('',#26257);
#7009=VERTEX_POINT('',#26259);
#7010=VERTEX_POINT('',#26261);
#7011=VERTEX_POINT('',#26263);
#7012=VERTEX_POINT('',#26265);
#7013=VERTEX_POINT('',#26267);
#7014=VERTEX_POINT('',#26269);
#7015=VERTEX_POINT('',#26271);
#7016=VERTEX_POINT('',#26273);
#7017=VERTEX_POINT('',#26275);
#7018=VERTEX_POINT('',#26277);
#7019=VERTEX_POINT('',#26279);
#7020=VERTEX_POINT('',#26281);
#7021=VERTEX_POINT('',#26283);
#7022=VERTEX_POINT('',#26285);
#7023=VERTEX_POINT('',#26287);
#7024=VERTEX_POINT('',#26289);
#7025=VERTEX_POINT('',#26291);
#7026=VERTEX_POINT('',#26293);
#7027=VERTEX_POINT('',#26295);
#7028=VERTEX_POINT('',#26297);
#7029=VERTEX_POINT('',#26299);
#7030=VERTEX_POINT('',#26301);
#7031=VERTEX_POINT('',#26303);
#7032=VERTEX_POINT('',#26305);
#7033=VERTEX_POINT('',#26307);
#7034=VERTEX_POINT('',#26309);
#7035=VERTEX_POINT('',#26311);
#7036=VERTEX_POINT('',#26313);
#7037=VERTEX_POINT('',#26315);
#7038=VERTEX_POINT('',#26317);
#7039=VERTEX_POINT('',#26319);
#7040=VERTEX_POINT('',#26321);
#7041=VERTEX_POINT('',#26323);
#7042=VERTEX_POINT('',#26325);
#7043=VERTEX_POINT('',#26327);
#7044=VERTEX_POINT('',#26329);
#7045=VERTEX_POINT('',#26331);
#7046=VERTEX_POINT('',#26333);
#7047=VERTEX_POINT('',#26335);
#7048=VERTEX_POINT('',#26337);
#7049=VERTEX_POINT('',#26339);
#7050=VERTEX_POINT('',#26341);
#7051=VERTEX_POINT('',#26343);
#7052=VERTEX_POINT('',#26347);
#7053=VERTEX_POINT('',#26352);
#7054=VERTEX_POINT('',#26354);
#7055=VERTEX_POINT('',#26355);
#7056=VERTEX_POINT('',#26357);
#7057=VERTEX_POINT('',#26359);
#7058=VERTEX_POINT('',#26361);
#7059=VERTEX_POINT('',#26363);
#7060=VERTEX_POINT('',#26365);
#7061=VERTEX_POINT('',#26367);
#7062=VERTEX_POINT('',#26369);
#7063=VERTEX_POINT('',#26371);
#7064=VERTEX_POINT('',#26373);
#7065=VERTEX_POINT('',#26375);
#7066=VERTEX_POINT('',#26377);
#7067=VERTEX_POINT('',#26379);
#7068=VERTEX_POINT('',#26381);
#7069=VERTEX_POINT('',#26383);
#7070=VERTEX_POINT('',#26385);
#7071=VERTEX_POINT('',#26387);
#7072=VERTEX_POINT('',#26389);
#7073=VERTEX_POINT('',#26391);
#7074=VERTEX_POINT('',#26393);
#7075=VERTEX_POINT('',#26395);
#7076=VERTEX_POINT('',#26397);
#7077=VERTEX_POINT('',#26399);
#7078=VERTEX_POINT('',#26401);
#7079=VERTEX_POINT('',#26403);
#7080=VERTEX_POINT('',#26405);
#7081=VERTEX_POINT('',#26407);
#7082=VERTEX_POINT('',#26409);
#7083=VERTEX_POINT('',#26411);
#7084=VERTEX_POINT('',#26413);
#7085=VERTEX_POINT('',#26415);
#7086=VERTEX_POINT('',#26417);
#7087=VERTEX_POINT('',#26419);
#7088=VERTEX_POINT('',#26421);
#7089=VERTEX_POINT('',#26423);
#7090=VERTEX_POINT('',#26425);
#7091=VERTEX_POINT('',#26427);
#7092=VERTEX_POINT('',#26429);
#7093=VERTEX_POINT('',#26431);
#7094=VERTEX_POINT('',#26433);
#7095=VERTEX_POINT('',#26435);
#7096=VERTEX_POINT('',#26437);
#7097=VERTEX_POINT('',#26439);
#7098=VERTEX_POINT('',#26441);
#7099=VERTEX_POINT('',#26443);
#7100=VERTEX_POINT('',#26445);
#7101=VERTEX_POINT('',#26447);
#7102=VERTEX_POINT('',#26449);
#7103=VERTEX_POINT('',#26451);
#7104=VERTEX_POINT('',#26453);
#7105=VERTEX_POINT('',#26455);
#7106=VERTEX_POINT('',#26457);
#7107=VERTEX_POINT('',#26459);
#7108=VERTEX_POINT('',#26461);
#7109=VERTEX_POINT('',#26463);
#7110=VERTEX_POINT('',#26465);
#7111=VERTEX_POINT('',#26467);
#7112=VERTEX_POINT('',#26469);
#7113=VERTEX_POINT('',#26471);
#7114=VERTEX_POINT('',#26473);
#7115=VERTEX_POINT('',#26475);
#7116=VERTEX_POINT('',#26477);
#7117=VERTEX_POINT('',#26479);
#7118=VERTEX_POINT('',#26481);
#7119=VERTEX_POINT('',#26483);
#7120=VERTEX_POINT('',#26485);
#7121=VERTEX_POINT('',#26487);
#7122=VERTEX_POINT('',#26489);
#7123=VERTEX_POINT('',#26491);
#7124=VERTEX_POINT('',#26493);
#7125=VERTEX_POINT('',#26495);
#7126=VERTEX_POINT('',#26497);
#7127=VERTEX_POINT('',#26499);
#7128=VERTEX_POINT('',#26501);
#7129=VERTEX_POINT('',#26503);
#7130=VERTEX_POINT('',#26505);
#7131=VERTEX_POINT('',#26507);
#7132=VERTEX_POINT('',#26509);
#7133=VERTEX_POINT('',#26511);
#7134=VERTEX_POINT('',#26515);
#8621=EDGE_CURVE('',#6945,#6946,#623,.T.);
#8622=EDGE_CURVE('',#6947,#6945,#624,.T.);
#8623=EDGE_CURVE('',#6946,#6947,#625,.T.);
#8624=EDGE_CURVE('',#6946,#6948,#4155,.T.);
#8625=EDGE_CURVE('',#6949,#6948,#626,.T.);
#8626=EDGE_CURVE('',#6950,#6949,#627,.T.);
#8627=EDGE_CURVE('',#6951,#6950,#628,.T.);
#8628=EDGE_CURVE('',#6948,#6951,#629,.T.);
#8629=EDGE_CURVE('',#6952,#6953,#630,.T.);
#8630=EDGE_CURVE('',#6953,#6952,#631,.T.);
#8631=EDGE_CURVE('',#6953,#6954,#4156,.T.);
#8632=EDGE_CURVE('',#6955,#6954,#632,.T.);
#8633=EDGE_CURVE('',#6956,#6955,#633,.T.);
#8634=EDGE_CURVE('',#6954,#6956,#634,.T.);
#8635=EDGE_CURVE('',#6957,#6957,#5773,.T.);
#8636=EDGE_CURVE('',#6957,#6947,#4157,.T.);
#8637=EDGE_CURVE('',#6945,#6958,#4158,.T.);
#8638=EDGE_CURVE('',#6958,#6958,#5774,.T.);
#8639=EDGE_CURVE('',#6959,#6960,#635,.T.);
#8640=EDGE_CURVE('',#6960,#6961,#636,.T.);
#8641=EDGE_CURVE('',#6961,#6959,#637,.T.);
#8642=EDGE_CURVE('',#6962,#6963,#638,.T.);
#8643=EDGE_CURVE('',#6963,#6964,#639,.T.);
#8644=EDGE_CURVE('',#6964,#6962,#640,.T.);
#8645=EDGE_CURVE('',#6961,#6965,#4159,.T.);
#8646=EDGE_CURVE('',#6966,#6965,#641,.T.);
#8647=EDGE_CURVE('',#6965,#6966,#642,.T.);
#8648=EDGE_CURVE('',#6967,#6968,#643,.T.);
#8649=EDGE_CURVE('',#6968,#6967,#644,.T.);
#8650=EDGE_CURVE('',#6968,#6964,#4160,.T.);
#8651=EDGE_CURVE('',#6969,#6969,#5775,.T.);
#8652=EDGE_CURVE('',#6969,#6949,#4161,.T.);
#8653=EDGE_CURVE('',#6951,#6970,#4162,.T.);
#8654=EDGE_CURVE('',#6970,#6970,#5776,.T.);
#8655=EDGE_CURVE('',#6971,#6971,#5777,.T.);
#8656=EDGE_CURVE('',#6972,#6973,#5778,.T.);
#8657=EDGE_CURVE('',#6974,#6973,#5779,.T.);
#8658=EDGE_CURVE('',#6974,#6975,#5780,.T.);
#8659=EDGE_CURVE('',#6976,#6975,#5781,.T.);
#8660=EDGE_CURVE('',#6976,#6977,#5782,.T.);
#8661=EDGE_CURVE('',#6978,#6977,#5783,.T.);
#8662=EDGE_CURVE('',#6978,#6979,#5784,.T.);
#8663=EDGE_CURVE('',#6980,#6979,#5785,.T.);
#8664=EDGE_CURVE('',#6980,#6981,#5786,.T.);
#8665=EDGE_CURVE('',#6982,#6981,#5787,.T.);
#8666=EDGE_CURVE('',#6982,#6983,#5788,.T.);
#8667=EDGE_CURVE('',#6984,#6983,#5789,.T.);
#8668=EDGE_CURVE('',#6984,#6985,#5790,.T.);
#8669=EDGE_CURVE('',#6986,#6985,#5791,.T.);
#8670=EDGE_CURVE('',#6986,#6987,#5792,.T.);
#8671=EDGE_CURVE('',#6988,#6987,#5793,.T.);
#8672=EDGE_CURVE('',#6988,#6989,#5794,.T.);
#8673=EDGE_CURVE('',#6990,#6989,#5795,.T.);
#8674=EDGE_CURVE('',#6990,#6991,#5796,.T.);
#8675=EDGE_CURVE('',#6992,#6991,#5797,.T.);
#8676=EDGE_CURVE('',#6992,#6993,#5798,.T.);
#8677=EDGE_CURVE('',#6994,#6993,#5799,.T.);
#8678=EDGE_CURVE('',#6994,#6995,#5800,.T.);
#8679=EDGE_CURVE('',#6996,#6995,#5801,.T.);
#8680=EDGE_CURVE('',#6996,#6997,#5802,.T.);
#8681=EDGE_CURVE('',#6998,#6997,#5803,.T.);
#8682=EDGE_CURVE('',#6998,#6999,#5804,.T.);
#8683=EDGE_CURVE('',#7000,#6999,#5805,.T.);
#8684=EDGE_CURVE('',#7000,#7001,#5806,.T.);
#8685=EDGE_CURVE('',#7002,#7001,#5807,.T.);
#8686=EDGE_CURVE('',#7002,#7003,#5808,.T.);
#8687=EDGE_CURVE('',#7004,#7003,#5809,.T.);
#8688=EDGE_CURVE('',#7004,#7005,#5810,.T.);
#8689=EDGE_CURVE('',#7006,#7005,#5811,.T.);
#8690=EDGE_CURVE('',#7006,#7007,#5812,.T.);
#8691=EDGE_CURVE('',#7008,#7007,#5813,.T.);
#8692=EDGE_CURVE('',#7008,#7009,#5814,.T.);
#8693=EDGE_CURVE('',#7010,#7009,#5815,.T.);
#8694=EDGE_CURVE('',#7010,#7011,#5816,.T.);
#8695=EDGE_CURVE('',#7012,#7011,#5817,.T.);
#8696=EDGE_CURVE('',#7012,#7013,#5818,.T.);
#8697=EDGE_CURVE('',#7014,#7013,#5819,.T.);
#8698=EDGE_CURVE('',#7014,#7015,#5820,.T.);
#8699=EDGE_CURVE('',#7016,#7015,#5821,.T.);
#8700=EDGE_CURVE('',#7016,#7017,#5822,.T.);
#8701=EDGE_CURVE('',#7018,#7017,#5823,.T.);
#8702=EDGE_CURVE('',#7018,#7019,#5824,.T.);
#8703=EDGE_CURVE('',#7020,#7019,#5825,.T.);
#8704=EDGE_CURVE('',#7020,#7021,#5826,.T.);
#8705=EDGE_CURVE('',#7022,#7021,#5827,.T.);
#8706=EDGE_CURVE('',#7022,#7023,#5828,.T.);
#8707=EDGE_CURVE('',#7024,#7023,#5829,.T.);
#8708=EDGE_CURVE('',#7024,#7025,#5830,.T.);
#8709=EDGE_CURVE('',#7026,#7025,#5831,.T.);
#8710=EDGE_CURVE('',#7026,#7027,#5832,.T.);
#8711=EDGE_CURVE('',#7028,#7027,#5833,.T.);
#8712=EDGE_CURVE('',#7028,#7029,#5834,.T.);
#8713=EDGE_CURVE('',#7030,#7029,#5835,.T.);
#8714=EDGE_CURVE('',#7030,#7031,#5836,.T.);
#8715=EDGE_CURVE('',#7032,#7031,#5837,.T.);
#8716=EDGE_CURVE('',#7032,#7033,#5838,.T.);
#8717=EDGE_CURVE('',#7034,#7033,#5839,.T.);
#8718=EDGE_CURVE('',#7034,#7035,#5840,.T.);
#8719=EDGE_CURVE('',#7036,#7035,#5841,.T.);
#8720=EDGE_CURVE('',#7036,#7037,#5842,.T.);
#8721=EDGE_CURVE('',#7038,#7037,#5843,.T.);
#8722=EDGE_CURVE('',#7038,#7039,#5844,.T.);
#8723=EDGE_CURVE('',#7040,#7039,#5845,.T.);
#8724=EDGE_CURVE('',#7040,#7041,#5846,.T.);
#8725=EDGE_CURVE('',#7042,#7041,#5847,.T.);
#8726=EDGE_CURVE('',#7042,#7043,#5848,.T.);
#8727=EDGE_CURVE('',#7044,#7043,#5849,.T.);
#8728=EDGE_CURVE('',#7044,#7045,#5850,.T.);
#8729=EDGE_CURVE('',#7046,#7045,#5851,.T.);
#8730=EDGE_CURVE('',#7046,#7047,#5852,.T.);
#8731=EDGE_CURVE('',#7048,#7047,#5853,.T.);
#8732=EDGE_CURVE('',#7048,#7049,#5854,.T.);
#8733=EDGE_CURVE('',#7050,#7049,#5855,.T.);
#8734=EDGE_CURVE('',#7050,#7051,#5856,.T.);
#8735=EDGE_CURVE('',#6972,#7051,#5857,.T.);
#8736=EDGE_CURVE('',#7052,#7052,#5858,.T.);
#8737=EDGE_CURVE('',#7052,#6971,#4163,.T.);
#8738=EDGE_CURVE('',#7053,#7053,#5859,.T.);
#8739=EDGE_CURVE('',#7054,#7055,#5860,.T.);
#8740=EDGE_CURVE('',#7055,#7056,#5861,.T.);
#8741=EDGE_CURVE('',#7056,#7057,#5862,.T.);
#8742=EDGE_CURVE('',#7057,#7058,#5863,.T.);
#8743=EDGE_CURVE('',#7058,#7059,#5864,.T.);
#8744=EDGE_CURVE('',#7059,#7060,#5865,.T.);
#8745=EDGE_CURVE('',#7060,#7061,#5866,.T.);
#8746=EDGE_CURVE('',#7061,#7062,#5867,.T.);
#8747=EDGE_CURVE('',#7062,#7063,#5868,.T.);
#8748=EDGE_CURVE('',#7063,#7064,#5869,.T.);
#8749=EDGE_CURVE('',#7064,#7065,#5870,.T.);
#8750=EDGE_CURVE('',#7065,#7066,#5871,.T.);
#8751=EDGE_CURVE('',#7066,#7067,#5872,.T.);
#8752=EDGE_CURVE('',#7067,#7068,#5873,.T.);
#8753=EDGE_CURVE('',#7068,#7069,#5874,.T.);
#8754=EDGE_CURVE('',#7069,#7070,#5875,.T.);
#8755=EDGE_CURVE('',#7070,#7071,#5876,.T.);
#8756=EDGE_CURVE('',#7071,#7072,#5877,.T.);
#8757=EDGE_CURVE('',#7072,#7073,#5878,.T.);
#8758=EDGE_CURVE('',#7073,#7074,#5879,.T.);
#8759=EDGE_CURVE('',#7074,#7075,#5880,.T.);
#8760=EDGE_CURVE('',#7075,#7076,#5881,.T.);
#8761=EDGE_CURVE('',#7076,#7077,#5882,.T.);
#8762=EDGE_CURVE('',#7077,#7078,#5883,.T.);
#8763=EDGE_CURVE('',#7078,#7079,#5884,.T.);
#8764=EDGE_CURVE('',#7079,#7080,#5885,.T.);
#8765=EDGE_CURVE('',#7080,#7081,#5886,.T.);
#8766=EDGE_CURVE('',#7081,#7082,#5887,.T.);
#8767=EDGE_CURVE('',#7082,#7083,#5888,.T.);
#8768=EDGE_CURVE('',#7083,#7084,#5889,.T.);
#8769=EDGE_CURVE('',#7084,#7085,#5890,.T.);
#8770=EDGE_CURVE('',#7085,#7086,#5891,.T.);
#8771=EDGE_CURVE('',#7086,#7087,#5892,.T.);
#8772=EDGE_CURVE('',#7087,#7088,#5893,.T.);
#8773=EDGE_CURVE('',#7088,#7089,#5894,.T.);
#8774=EDGE_CURVE('',#7089,#7090,#5895,.T.);
#8775=EDGE_CURVE('',#7090,#7091,#5896,.T.);
#8776=EDGE_CURVE('',#7091,#7092,#5897,.T.);
#8777=EDGE_CURVE('',#7092,#7093,#5898,.T.);
#8778=EDGE_CURVE('',#7093,#7094,#5899,.T.);
#8779=EDGE_CURVE('',#7094,#7095,#5900,.T.);
#8780=EDGE_CURVE('',#7095,#7096,#5901,.T.);
#8781=EDGE_CURVE('',#7096,#7097,#5902,.T.);
#8782=EDGE_CURVE('',#7097,#7098,#5903,.T.);
#8783=EDGE_CURVE('',#7098,#7099,#5904,.T.);
#8784=EDGE_CURVE('',#7099,#7100,#5905,.T.);
#8785=EDGE_CURVE('',#7100,#7101,#5906,.T.);
#8786=EDGE_CURVE('',#7101,#7102,#5907,.T.);
#8787=EDGE_CURVE('',#7102,#7103,#5908,.T.);
#8788=EDGE_CURVE('',#7103,#7104,#5909,.T.);
#8789=EDGE_CURVE('',#7104,#7105,#5910,.T.);
#8790=EDGE_CURVE('',#7105,#7106,#5911,.T.);
#8791=EDGE_CURVE('',#7106,#7107,#5912,.T.);
#8792=EDGE_CURVE('',#7107,#7108,#5913,.T.);
#8793=EDGE_CURVE('',#7108,#7109,#5914,.T.);
#8794=EDGE_CURVE('',#7109,#7110,#5915,.T.);
#8795=EDGE_CURVE('',#7110,#7111,#5916,.T.);
#8796=EDGE_CURVE('',#7111,#7112,#5917,.T.);
#8797=EDGE_CURVE('',#7112,#7113,#5918,.T.);
#8798=EDGE_CURVE('',#7113,#7114,#5919,.T.);
#8799=EDGE_CURVE('',#7114,#7115,#5920,.T.);
#8800=EDGE_CURVE('',#7115,#7116,#5921,.T.);
#8801=EDGE_CURVE('',#7116,#7117,#5922,.T.);
#8802=EDGE_CURVE('',#7117,#7118,#5923,.T.);
#8803=EDGE_CURVE('',#7118,#7119,#5924,.T.);
#8804=EDGE_CURVE('',#7119,#7120,#5925,.T.);
#8805=EDGE_CURVE('',#7120,#7121,#5926,.T.);
#8806=EDGE_CURVE('',#7121,#7122,#5927,.T.);
#8807=EDGE_CURVE('',#7122,#7123,#5928,.T.);
#8808=EDGE_CURVE('',#7123,#7124,#5929,.T.);
#8809=EDGE_CURVE('',#7124,#7125,#5930,.T.);
#8810=EDGE_CURVE('',#7125,#7126,#5931,.T.);
#8811=EDGE_CURVE('',#7126,#7127,#5932,.T.);
#8812=EDGE_CURVE('',#7127,#7128,#5933,.T.);
#8813=EDGE_CURVE('',#7128,#7129,#5934,.T.);
#8814=EDGE_CURVE('',#7129,#7130,#5935,.T.);
#8815=EDGE_CURVE('',#7130,#7131,#5936,.T.);
#8816=EDGE_CURVE('',#7131,#7132,#5937,.T.);
#8817=EDGE_CURVE('',#7132,#7133,#5938,.T.);
#8818=EDGE_CURVE('',#7133,#7054,#5939,.T.);
#8819=EDGE_CURVE('',#7134,#7134,#5940,.T.);
#8820=EDGE_CURVE('',#7134,#7053,#4164,.T.);
#8821=EDGE_CURVE('',#7055,#6972,#4165,.T.);
#8822=EDGE_CURVE('',#6973,#7054,#4166,.T.);
#8823=EDGE_CURVE('',#7133,#6974,#4167,.T.);
#8824=EDGE_CURVE('',#6975,#7132,#4168,.T.);
#8825=EDGE_CURVE('',#7131,#6976,#4169,.T.);
#8826=EDGE_CURVE('',#6977,#7130,#4170,.T.);
#8827=EDGE_CURVE('',#7129,#6978,#4171,.T.);
#8828=EDGE_CURVE('',#6979,#7128,#4172,.T.);
#8829=EDGE_CURVE('',#7127,#6980,#4173,.T.);
#8830=EDGE_CURVE('',#6981,#7126,#4174,.T.);
#8831=EDGE_CURVE('',#7125,#6982,#4175,.T.);
#8832=EDGE_CURVE('',#6983,#7124,#4176,.T.);
#8833=EDGE_CURVE('',#7123,#6984,#4177,.T.);
#8834=EDGE_CURVE('',#6985,#7122,#4178,.T.);
#8835=EDGE_CURVE('',#7121,#6986,#4179,.T.);
#8836=EDGE_CURVE('',#6987,#7120,#4180,.T.);
#8837=EDGE_CURVE('',#7119,#6988,#4181,.T.);
#8838=EDGE_CURVE('',#6989,#7118,#4182,.T.);
#8839=EDGE_CURVE('',#7117,#6990,#4183,.T.);
#8840=EDGE_CURVE('',#6991,#7116,#4184,.T.);
#8841=EDGE_CURVE('',#7115,#6992,#4185,.T.);
#8842=EDGE_CURVE('',#6993,#7114,#4186,.T.);
#8843=EDGE_CURVE('',#7113,#6994,#4187,.T.);
#8844=EDGE_CURVE('',#6995,#7112,#4188,.T.);
#8845=EDGE_CURVE('',#7111,#6996,#4189,.T.);
#8846=EDGE_CURVE('',#6997,#7110,#4190,.T.);
#8847=EDGE_CURVE('',#7109,#6998,#4191,.T.);
#8848=EDGE_CURVE('',#6999,#7108,#4192,.T.);
#8849=EDGE_CURVE('',#7107,#7000,#4193,.T.);
#8850=EDGE_CURVE('',#7001,#7106,#4194,.T.);
#8851=EDGE_CURVE('',#7105,#7002,#4195,.T.);
#8852=EDGE_CURVE('',#7003,#7104,#4196,.T.);
#8853=EDGE_CURVE('',#7103,#7004,#4197,.T.);
#8854=EDGE_CURVE('',#7005,#7102,#4198,.T.);
#8855=EDGE_CURVE('',#7101,#7006,#4199,.T.);
#8856=EDGE_CURVE('',#7007,#7100,#4200,.T.);
#8857=EDGE_CURVE('',#7099,#7008,#4201,.T.);
#8858=EDGE_CURVE('',#7009,#7098,#4202,.T.);
#8859=EDGE_CURVE('',#7097,#7010,#4203,.T.);
#8860=EDGE_CURVE('',#7011,#7096,#4204,.T.);
#8861=EDGE_CURVE('',#7095,#7012,#4205,.T.);
#8862=EDGE_CURVE('',#7013,#7094,#4206,.T.);
#8863=EDGE_CURVE('',#7093,#7014,#4207,.T.);
#8864=EDGE_CURVE('',#7015,#7092,#4208,.T.);
#8865=EDGE_CURVE('',#7091,#7016,#4209,.T.);
#8866=EDGE_CURVE('',#7017,#7090,#4210,.T.);
#8867=EDGE_CURVE('',#7089,#7018,#4211,.T.);
#8868=EDGE_CURVE('',#7019,#7088,#4212,.T.);
#8869=EDGE_CURVE('',#7087,#7020,#4213,.T.);
#8870=EDGE_CURVE('',#7021,#7086,#4214,.T.);
#8871=EDGE_CURVE('',#7085,#7022,#4215,.T.);
#8872=EDGE_CURVE('',#7023,#7084,#4216,.T.);
#8873=EDGE_CURVE('',#7083,#7024,#4217,.T.);
#8874=EDGE_CURVE('',#7025,#7082,#4218,.T.);
#8875=EDGE_CURVE('',#7081,#7026,#4219,.T.);
#8876=EDGE_CURVE('',#7027,#7080,#4220,.T.);
#8877=EDGE_CURVE('',#7079,#7028,#4221,.T.);
#8878=EDGE_CURVE('',#7029,#7078,#4222,.T.);
#8879=EDGE_CURVE('',#7077,#7030,#4223,.T.);
#8880=EDGE_CURVE('',#7031,#7076,#4224,.T.);
#8881=EDGE_CURVE('',#7075,#7032,#4225,.T.);
#8882=EDGE_CURVE('',#7033,#7074,#4226,.T.);
#8883=EDGE_CURVE('',#7073,#7034,#4227,.T.);
#8884=EDGE_CURVE('',#7035,#7072,#4228,.T.);
#8885=EDGE_CURVE('',#7071,#7036,#4229,.T.);
#8886=EDGE_CURVE('',#7037,#7070,#4230,.T.);
#8887=EDGE_CURVE('',#7069,#7038,#4231,.T.);
#8888=EDGE_CURVE('',#7039,#7068,#4232,.T.);
#8889=EDGE_CURVE('',#7067,#7040,#4233,.T.);
#8890=EDGE_CURVE('',#7041,#7066,#4234,.T.);
#8891=EDGE_CURVE('',#7065,#7042,#4235,.T.);
#8892=EDGE_CURVE('',#7043,#7064,#4236,.T.);
#8893=EDGE_CURVE('',#7063,#7044,#4237,.T.);
#8894=EDGE_CURVE('',#7045,#7062,#4238,.T.);
#8895=EDGE_CURVE('',#7061,#7046,#4239,.T.);
#8896=EDGE_CURVE('',#7047,#7060,#4240,.T.);
#8897=EDGE_CURVE('',#7059,#7048,#4241,.T.);
#8898=EDGE_CURVE('',#7049,#7058,#4242,.T.);
#8899=EDGE_CURVE('',#7051,#7056,#4243,.T.);
#8900=EDGE_CURVE('',#7057,#7050,#4244,.T.);
#11858=ORIENTED_EDGE('',*,*,#8621,.F.);
#11859=ORIENTED_EDGE('',*,*,#8622,.F.);
#11860=ORIENTED_EDGE('',*,*,#8623,.F.);
#11861=ORIENTED_EDGE('',*,*,#8624,.T.);
#11862=ORIENTED_EDGE('',*,*,#8625,.F.);
#11863=ORIENTED_EDGE('',*,*,#8626,.F.);
#11864=ORIENTED_EDGE('',*,*,#8627,.F.);
#11865=ORIENTED_EDGE('',*,*,#8628,.F.);
#11866=ORIENTED_EDGE('',*,*,#8624,.F.);
#11867=ORIENTED_EDGE('',*,*,#8629,.F.);
#11868=ORIENTED_EDGE('',*,*,#8630,.F.);
#11869=ORIENTED_EDGE('',*,*,#8631,.T.);
#11870=ORIENTED_EDGE('',*,*,#8632,.F.);
#11871=ORIENTED_EDGE('',*,*,#8633,.F.);
#11872=ORIENTED_EDGE('',*,*,#8634,.F.);
#11873=ORIENTED_EDGE('',*,*,#8631,.F.);
#11874=ORIENTED_EDGE('',*,*,#8635,.F.);
#11875=ORIENTED_EDGE('',*,*,#8636,.T.);
#11876=ORIENTED_EDGE('',*,*,#8622,.T.);
#11877=ORIENTED_EDGE('',*,*,#8637,.T.);
#11878=ORIENTED_EDGE('',*,*,#8638,.F.);
#11879=ORIENTED_EDGE('',*,*,#8637,.F.);
#11880=ORIENTED_EDGE('',*,*,#8621,.T.);
#11881=ORIENTED_EDGE('',*,*,#8623,.T.);
#11882=ORIENTED_EDGE('',*,*,#8636,.F.);
#11883=ORIENTED_EDGE('',*,*,#8633,.T.);
#11884=ORIENTED_EDGE('',*,*,#8632,.T.);
#11885=ORIENTED_EDGE('',*,*,#8634,.T.);
#11886=ORIENTED_EDGE('',*,*,#8639,.T.);
#11887=ORIENTED_EDGE('',*,*,#8640,.T.);
#11888=ORIENTED_EDGE('',*,*,#8641,.T.);
#11889=ORIENTED_EDGE('',*,*,#8642,.T.);
#11890=ORIENTED_EDGE('',*,*,#8643,.T.);
#11891=ORIENTED_EDGE('',*,*,#8644,.T.);
#11892=ORIENTED_EDGE('',*,*,#8640,.F.);
#11893=ORIENTED_EDGE('',*,*,#8639,.F.);
#11894=ORIENTED_EDGE('',*,*,#8641,.F.);
#11895=ORIENTED_EDGE('',*,*,#8645,.T.);
#11896=ORIENTED_EDGE('',*,*,#8646,.F.);
#11897=ORIENTED_EDGE('',*,*,#8647,.F.);
#11898=ORIENTED_EDGE('',*,*,#8645,.F.);
#11899=ORIENTED_EDGE('',*,*,#8648,.F.);
#11900=ORIENTED_EDGE('',*,*,#8649,.F.);
#11901=ORIENTED_EDGE('',*,*,#8650,.T.);
#11902=ORIENTED_EDGE('',*,*,#8643,.F.);
#11903=ORIENTED_EDGE('',*,*,#8642,.F.);
#11904=ORIENTED_EDGE('',*,*,#8644,.F.);
#11905=ORIENTED_EDGE('',*,*,#8650,.F.);
#11906=ORIENTED_EDGE('',*,*,#8651,.F.);
#11907=ORIENTED_EDGE('',*,*,#8652,.T.);
#11908=ORIENTED_EDGE('',*,*,#8625,.T.);
#11909=ORIENTED_EDGE('',*,*,#8628,.T.);
#11910=ORIENTED_EDGE('',*,*,#8653,.T.);
#11911=ORIENTED_EDGE('',*,*,#8654,.F.);
#11912=ORIENTED_EDGE('',*,*,#8653,.F.);
#11913=ORIENTED_EDGE('',*,*,#8627,.T.);
#11914=ORIENTED_EDGE('',*,*,#8626,.T.);
#11915=ORIENTED_EDGE('',*,*,#8652,.F.);
#11916=ORIENTED_EDGE('',*,*,#8629,.T.);
#11917=ORIENTED_EDGE('',*,*,#8630,.T.);
#11918=ORIENTED_EDGE('',*,*,#8648,.T.);
#11919=ORIENTED_EDGE('',*,*,#8649,.T.);
#11920=ORIENTED_EDGE('',*,*,#8646,.T.);
#11921=ORIENTED_EDGE('',*,*,#8647,.T.);
#11922=ORIENTED_EDGE('',*,*,#8635,.T.);
#11923=ORIENTED_EDGE('',*,*,#8651,.T.);
#11924=ORIENTED_EDGE('',*,*,#8655,.T.);
#11925=ORIENTED_EDGE('',*,*,#8656,.T.);
#11926=ORIENTED_EDGE('',*,*,#8657,.F.);
#11927=ORIENTED_EDGE('',*,*,#8658,.T.);
#11928=ORIENTED_EDGE('',*,*,#8659,.F.);
#11929=ORIENTED_EDGE('',*,*,#8660,.T.);
#11930=ORIENTED_EDGE('',*,*,#8661,.F.);
#11931=ORIENTED_EDGE('',*,*,#8662,.T.);
#11932=ORIENTED_EDGE('',*,*,#8663,.F.);
#11933=ORIENTED_EDGE('',*,*,#8664,.T.);
#11934=ORIENTED_EDGE('',*,*,#8665,.F.);
#11935=ORIENTED_EDGE('',*,*,#8666,.T.);
#11936=ORIENTED_EDGE('',*,*,#8667,.F.);
#11937=ORIENTED_EDGE('',*,*,#8668,.T.);
#11938=ORIENTED_EDGE('',*,*,#8669,.F.);
#11939=ORIENTED_EDGE('',*,*,#8670,.T.);
#11940=ORIENTED_EDGE('',*,*,#8671,.F.);
#11941=ORIENTED_EDGE('',*,*,#8672,.T.);
#11942=ORIENTED_EDGE('',*,*,#8673,.F.);
#11943=ORIENTED_EDGE('',*,*,#8674,.T.);
#11944=ORIENTED_EDGE('',*,*,#8675,.F.);
#11945=ORIENTED_EDGE('',*,*,#8676,.T.);
#11946=ORIENTED_EDGE('',*,*,#8677,.F.);
#11947=ORIENTED_EDGE('',*,*,#8678,.T.);
#11948=ORIENTED_EDGE('',*,*,#8679,.F.);
#11949=ORIENTED_EDGE('',*,*,#8680,.T.);
#11950=ORIENTED_EDGE('',*,*,#8681,.F.);
#11951=ORIENTED_EDGE('',*,*,#8682,.T.);
#11952=ORIENTED_EDGE('',*,*,#8683,.F.);
#11953=ORIENTED_EDGE('',*,*,#8684,.T.);
#11954=ORIENTED_EDGE('',*,*,#8685,.F.);
#11955=ORIENTED_EDGE('',*,*,#8686,.T.);
#11956=ORIENTED_EDGE('',*,*,#8687,.F.);
#11957=ORIENTED_EDGE('',*,*,#8688,.T.);
#11958=ORIENTED_EDGE('',*,*,#8689,.F.);
#11959=ORIENTED_EDGE('',*,*,#8690,.T.);
#11960=ORIENTED_EDGE('',*,*,#8691,.F.);
#11961=ORIENTED_EDGE('',*,*,#8692,.T.);
#11962=ORIENTED_EDGE('',*,*,#8693,.F.);
#11963=ORIENTED_EDGE('',*,*,#8694,.T.);
#11964=ORIENTED_EDGE('',*,*,#8695,.F.);
#11965=ORIENTED_EDGE('',*,*,#8696,.T.);
#11966=ORIENTED_EDGE('',*,*,#8697,.F.);
#11967=ORIENTED_EDGE('',*,*,#8698,.T.);
#11968=ORIENTED_EDGE('',*,*,#8699,.F.);
#11969=ORIENTED_EDGE('',*,*,#8700,.T.);
#11970=ORIENTED_EDGE('',*,*,#8701,.F.);
#11971=ORIENTED_EDGE('',*,*,#8702,.T.);
#11972=ORIENTED_EDGE('',*,*,#8703,.F.);
#11973=ORIENTED_EDGE('',*,*,#8704,.T.);
#11974=ORIENTED_EDGE('',*,*,#8705,.F.);
#11975=ORIENTED_EDGE('',*,*,#8706,.T.);
#11976=ORIENTED_EDGE('',*,*,#8707,.F.);
#11977=ORIENTED_EDGE('',*,*,#8708,.T.);
#11978=ORIENTED_EDGE('',*,*,#8709,.F.);
#11979=ORIENTED_EDGE('',*,*,#8710,.T.);
#11980=ORIENTED_EDGE('',*,*,#8711,.F.);
#11981=ORIENTED_EDGE('',*,*,#8712,.T.);
#11982=ORIENTED_EDGE('',*,*,#8713,.F.);
#11983=ORIENTED_EDGE('',*,*,#8714,.T.);
#11984=ORIENTED_EDGE('',*,*,#8715,.F.);
#11985=ORIENTED_EDGE('',*,*,#8716,.T.);
#11986=ORIENTED_EDGE('',*,*,#8717,.F.);
#11987=ORIENTED_EDGE('',*,*,#8718,.T.);
#11988=ORIENTED_EDGE('',*,*,#8719,.F.);
#11989=ORIENTED_EDGE('',*,*,#8720,.T.);
#11990=ORIENTED_EDGE('',*,*,#8721,.F.);
#11991=ORIENTED_EDGE('',*,*,#8722,.T.);
#11992=ORIENTED_EDGE('',*,*,#8723,.F.);
#11993=ORIENTED_EDGE('',*,*,#8724,.T.);
#11994=ORIENTED_EDGE('',*,*,#8725,.F.);
#11995=ORIENTED_EDGE('',*,*,#8726,.T.);
#11996=ORIENTED_EDGE('',*,*,#8727,.F.);
#11997=ORIENTED_EDGE('',*,*,#8728,.T.);
#11998=ORIENTED_EDGE('',*,*,#8729,.F.);
#11999=ORIENTED_EDGE('',*,*,#8730,.T.);
#12000=ORIENTED_EDGE('',*,*,#8731,.F.);
#12001=ORIENTED_EDGE('',*,*,#8732,.T.);
#12002=ORIENTED_EDGE('',*,*,#8733,.F.);
#12003=ORIENTED_EDGE('',*,*,#8734,.T.);
#12004=ORIENTED_EDGE('',*,*,#8735,.F.);
#12005=ORIENTED_EDGE('',*,*,#8736,.F.);
#12006=ORIENTED_EDGE('',*,*,#8737,.T.);
#12007=ORIENTED_EDGE('',*,*,#8655,.F.);
#12008=ORIENTED_EDGE('',*,*,#8737,.F.);
#12009=ORIENTED_EDGE('',*,*,#8736,.T.);
#12010=ORIENTED_EDGE('',*,*,#8638,.T.);
#12011=ORIENTED_EDGE('',*,*,#8738,.F.);
#12012=ORIENTED_EDGE('',*,*,#8739,.T.);
#12013=ORIENTED_EDGE('',*,*,#8740,.T.);
#12014=ORIENTED_EDGE('',*,*,#8741,.T.);
#12015=ORIENTED_EDGE('',*,*,#8742,.T.);
#12016=ORIENTED_EDGE('',*,*,#8743,.T.);
#12017=ORIENTED_EDGE('',*,*,#8744,.T.);
#12018=ORIENTED_EDGE('',*,*,#8745,.T.);
#12019=ORIENTED_EDGE('',*,*,#8746,.T.);
#12020=ORIENTED_EDGE('',*,*,#8747,.T.);
#12021=ORIENTED_EDGE('',*,*,#8748,.T.);
#12022=ORIENTED_EDGE('',*,*,#8749,.T.);
#12023=ORIENTED_EDGE('',*,*,#8750,.T.);
#12024=ORIENTED_EDGE('',*,*,#8751,.T.);
#12025=ORIENTED_EDGE('',*,*,#8752,.T.);
#12026=ORIENTED_EDGE('',*,*,#8753,.T.);
#12027=ORIENTED_EDGE('',*,*,#8754,.T.);
#12028=ORIENTED_EDGE('',*,*,#8755,.T.);
#12029=ORIENTED_EDGE('',*,*,#8756,.T.);
#12030=ORIENTED_EDGE('',*,*,#8757,.T.);
#12031=ORIENTED_EDGE('',*,*,#8758,.T.);
#12032=ORIENTED_EDGE('',*,*,#8759,.T.);
#12033=ORIENTED_EDGE('',*,*,#8760,.T.);
#12034=ORIENTED_EDGE('',*,*,#8761,.T.);
#12035=ORIENTED_EDGE('',*,*,#8762,.T.);
#12036=ORIENTED_EDGE('',*,*,#8763,.T.);
#12037=ORIENTED_EDGE('',*,*,#8764,.T.);
#12038=ORIENTED_EDGE('',*,*,#8765,.T.);
#12039=ORIENTED_EDGE('',*,*,#8766,.T.);
#12040=ORIENTED_EDGE('',*,*,#8767,.T.);
#12041=ORIENTED_EDGE('',*,*,#8768,.T.);
#12042=ORIENTED_EDGE('',*,*,#8769,.T.);
#12043=ORIENTED_EDGE('',*,*,#8770,.T.);
#12044=ORIENTED_EDGE('',*,*,#8771,.T.);
#12045=ORIENTED_EDGE('',*,*,#8772,.T.);
#12046=ORIENTED_EDGE('',*,*,#8773,.T.);
#12047=ORIENTED_EDGE('',*,*,#8774,.T.);
#12048=ORIENTED_EDGE('',*,*,#8775,.T.);
#12049=ORIENTED_EDGE('',*,*,#8776,.T.);
#12050=ORIENTED_EDGE('',*,*,#8777,.T.);
#12051=ORIENTED_EDGE('',*,*,#8778,.T.);
#12052=ORIENTED_EDGE('',*,*,#8779,.T.);
#12053=ORIENTED_EDGE('',*,*,#8780,.T.);
#12054=ORIENTED_EDGE('',*,*,#8781,.T.);
#12055=ORIENTED_EDGE('',*,*,#8782,.T.);
#12056=ORIENTED_EDGE('',*,*,#8783,.T.);
#12057=ORIENTED_EDGE('',*,*,#8784,.T.);
#12058=ORIENTED_EDGE('',*,*,#8785,.T.);
#12059=ORIENTED_EDGE('',*,*,#8786,.T.);
#12060=ORIENTED_EDGE('',*,*,#8787,.T.);
#12061=ORIENTED_EDGE('',*,*,#8788,.T.);
#12062=ORIENTED_EDGE('',*,*,#8789,.T.);
#12063=ORIENTED_EDGE('',*,*,#8790,.T.);
#12064=ORIENTED_EDGE('',*,*,#8791,.T.);
#12065=ORIENTED_EDGE('',*,*,#8792,.T.);
#12066=ORIENTED_EDGE('',*,*,#8793,.T.);
#12067=ORIENTED_EDGE('',*,*,#8794,.T.);
#12068=ORIENTED_EDGE('',*,*,#8795,.T.);
#12069=ORIENTED_EDGE('',*,*,#8796,.T.);
#12070=ORIENTED_EDGE('',*,*,#8797,.T.);
#12071=ORIENTED_EDGE('',*,*,#8798,.T.);
#12072=ORIENTED_EDGE('',*,*,#8799,.T.);
#12073=ORIENTED_EDGE('',*,*,#8800,.T.);
#12074=ORIENTED_EDGE('',*,*,#8801,.T.);
#12075=ORIENTED_EDGE('',*,*,#8802,.T.);
#12076=ORIENTED_EDGE('',*,*,#8803,.T.);
#12077=ORIENTED_EDGE('',*,*,#8804,.T.);
#12078=ORIENTED_EDGE('',*,*,#8805,.T.);
#12079=ORIENTED_EDGE('',*,*,#8806,.T.);
#12080=ORIENTED_EDGE('',*,*,#8807,.T.);
#12081=ORIENTED_EDGE('',*,*,#8808,.T.);
#12082=ORIENTED_EDGE('',*,*,#8809,.T.);
#12083=ORIENTED_EDGE('',*,*,#8810,.T.);
#12084=ORIENTED_EDGE('',*,*,#8811,.T.);
#12085=ORIENTED_EDGE('',*,*,#8812,.T.);
#12086=ORIENTED_EDGE('',*,*,#8813,.T.);
#12087=ORIENTED_EDGE('',*,*,#8814,.T.);
#12088=ORIENTED_EDGE('',*,*,#8815,.T.);
#12089=ORIENTED_EDGE('',*,*,#8816,.T.);
#12090=ORIENTED_EDGE('',*,*,#8817,.T.);
#12091=ORIENTED_EDGE('',*,*,#8818,.T.);
#12092=ORIENTED_EDGE('',*,*,#8819,.F.);
#12093=ORIENTED_EDGE('',*,*,#8820,.T.);
#12094=ORIENTED_EDGE('',*,*,#8738,.T.);
#12095=ORIENTED_EDGE('',*,*,#8820,.F.);
#12096=ORIENTED_EDGE('',*,*,#8819,.T.);
#12097=ORIENTED_EDGE('',*,*,#8654,.T.);
#12098=ORIENTED_EDGE('',*,*,#8821,.F.);
#12099=ORIENTED_EDGE('',*,*,#8739,.F.);
#12100=ORIENTED_EDGE('',*,*,#8822,.F.);
#12101=ORIENTED_EDGE('',*,*,#8656,.F.);
#12102=ORIENTED_EDGE('',*,*,#8822,.T.);
#12103=ORIENTED_EDGE('',*,*,#8818,.F.);
#12104=ORIENTED_EDGE('',*,*,#8823,.T.);
#12105=ORIENTED_EDGE('',*,*,#8657,.T.);
#12106=ORIENTED_EDGE('',*,*,#8823,.F.);
#12107=ORIENTED_EDGE('',*,*,#8817,.F.);
#12108=ORIENTED_EDGE('',*,*,#8824,.F.);
#12109=ORIENTED_EDGE('',*,*,#8658,.F.);
#12110=ORIENTED_EDGE('',*,*,#8824,.T.);
#12111=ORIENTED_EDGE('',*,*,#8816,.F.);
#12112=ORIENTED_EDGE('',*,*,#8825,.T.);
#12113=ORIENTED_EDGE('',*,*,#8659,.T.);
#12114=ORIENTED_EDGE('',*,*,#8825,.F.);
#12115=ORIENTED_EDGE('',*,*,#8815,.F.);
#12116=ORIENTED_EDGE('',*,*,#8826,.F.);
#12117=ORIENTED_EDGE('',*,*,#8660,.F.);
#12118=ORIENTED_EDGE('',*,*,#8826,.T.);
#12119=ORIENTED_EDGE('',*,*,#8814,.F.);
#12120=ORIENTED_EDGE('',*,*,#8827,.T.);
#12121=ORIENTED_EDGE('',*,*,#8661,.T.);
#12122=ORIENTED_EDGE('',*,*,#8827,.F.);
#12123=ORIENTED_EDGE('',*,*,#8813,.F.);
#12124=ORIENTED_EDGE('',*,*,#8828,.F.);
#12125=ORIENTED_EDGE('',*,*,#8662,.F.);
#12126=ORIENTED_EDGE('',*,*,#8828,.T.);
#12127=ORIENTED_EDGE('',*,*,#8812,.F.);
#12128=ORIENTED_EDGE('',*,*,#8829,.T.);
#12129=ORIENTED_EDGE('',*,*,#8663,.T.);
#12130=ORIENTED_EDGE('',*,*,#8829,.F.);
#12131=ORIENTED_EDGE('',*,*,#8811,.F.);
#12132=ORIENTED_EDGE('',*,*,#8830,.F.);
#12133=ORIENTED_EDGE('',*,*,#8664,.F.);
#12134=ORIENTED_EDGE('',*,*,#8830,.T.);
#12135=ORIENTED_EDGE('',*,*,#8810,.F.);
#12136=ORIENTED_EDGE('',*,*,#8831,.T.);
#12137=ORIENTED_EDGE('',*,*,#8665,.T.);
#12138=ORIENTED_EDGE('',*,*,#8831,.F.);
#12139=ORIENTED_EDGE('',*,*,#8809,.F.);
#12140=ORIENTED_EDGE('',*,*,#8832,.F.);
#12141=ORIENTED_EDGE('',*,*,#8666,.F.);
#12142=ORIENTED_EDGE('',*,*,#8832,.T.);
#12143=ORIENTED_EDGE('',*,*,#8808,.F.);
#12144=ORIENTED_EDGE('',*,*,#8833,.T.);
#12145=ORIENTED_EDGE('',*,*,#8667,.T.);
#12146=ORIENTED_EDGE('',*,*,#8833,.F.);
#12147=ORIENTED_EDGE('',*,*,#8807,.F.);
#12148=ORIENTED_EDGE('',*,*,#8834,.F.);
#12149=ORIENTED_EDGE('',*,*,#8668,.F.);
#12150=ORIENTED_EDGE('',*,*,#8834,.T.);
#12151=ORIENTED_EDGE('',*,*,#8806,.F.);
#12152=ORIENTED_EDGE('',*,*,#8835,.T.);
#12153=ORIENTED_EDGE('',*,*,#8669,.T.);
#12154=ORIENTED_EDGE('',*,*,#8835,.F.);
#12155=ORIENTED_EDGE('',*,*,#8805,.F.);
#12156=ORIENTED_EDGE('',*,*,#8836,.F.);
#12157=ORIENTED_EDGE('',*,*,#8670,.F.);
#12158=ORIENTED_EDGE('',*,*,#8836,.T.);
#12159=ORIENTED_EDGE('',*,*,#8804,.F.);
#12160=ORIENTED_EDGE('',*,*,#8837,.T.);
#12161=ORIENTED_EDGE('',*,*,#8671,.T.);
#12162=ORIENTED_EDGE('',*,*,#8837,.F.);
#12163=ORIENTED_EDGE('',*,*,#8803,.F.);
#12164=ORIENTED_EDGE('',*,*,#8838,.F.);
#12165=ORIENTED_EDGE('',*,*,#8672,.F.);
#12166=ORIENTED_EDGE('',*,*,#8838,.T.);
#12167=ORIENTED_EDGE('',*,*,#8802,.F.);
#12168=ORIENTED_EDGE('',*,*,#8839,.T.);
#12169=ORIENTED_EDGE('',*,*,#8673,.T.);
#12170=ORIENTED_EDGE('',*,*,#8839,.F.);
#12171=ORIENTED_EDGE('',*,*,#8801,.F.);
#12172=ORIENTED_EDGE('',*,*,#8840,.F.);
#12173=ORIENTED_EDGE('',*,*,#8674,.F.);
#12174=ORIENTED_EDGE('',*,*,#8840,.T.);
#12175=ORIENTED_EDGE('',*,*,#8800,.F.);
#12176=ORIENTED_EDGE('',*,*,#8841,.T.);
#12177=ORIENTED_EDGE('',*,*,#8675,.T.);
#12178=ORIENTED_EDGE('',*,*,#8841,.F.);
#12179=ORIENTED_EDGE('',*,*,#8799,.F.);
#12180=ORIENTED_EDGE('',*,*,#8842,.F.);
#12181=ORIENTED_EDGE('',*,*,#8676,.F.);
#12182=ORIENTED_EDGE('',*,*,#8842,.T.);
#12183=ORIENTED_EDGE('',*,*,#8798,.F.);
#12184=ORIENTED_EDGE('',*,*,#8843,.T.);
#12185=ORIENTED_EDGE('',*,*,#8677,.T.);
#12186=ORIENTED_EDGE('',*,*,#8843,.F.);
#12187=ORIENTED_EDGE('',*,*,#8797,.F.);
#12188=ORIENTED_EDGE('',*,*,#8844,.F.);
#12189=ORIENTED_EDGE('',*,*,#8678,.F.);
#12190=ORIENTED_EDGE('',*,*,#8844,.T.);
#12191=ORIENTED_EDGE('',*,*,#8796,.F.);
#12192=ORIENTED_EDGE('',*,*,#8845,.T.);
#12193=ORIENTED_EDGE('',*,*,#8679,.T.);
#12194=ORIENTED_EDGE('',*,*,#8845,.F.);
#12195=ORIENTED_EDGE('',*,*,#8795,.F.);
#12196=ORIENTED_EDGE('',*,*,#8846,.F.);
#12197=ORIENTED_EDGE('',*,*,#8680,.F.);
#12198=ORIENTED_EDGE('',*,*,#8846,.T.);
#12199=ORIENTED_EDGE('',*,*,#8794,.F.);
#12200=ORIENTED_EDGE('',*,*,#8847,.T.);
#12201=ORIENTED_EDGE('',*,*,#8681,.T.);
#12202=ORIENTED_EDGE('',*,*,#8847,.F.);
#12203=ORIENTED_EDGE('',*,*,#8793,.F.);
#12204=ORIENTED_EDGE('',*,*,#8848,.F.);
#12205=ORIENTED_EDGE('',*,*,#8682,.F.);
#12206=ORIENTED_EDGE('',*,*,#8848,.T.);
#12207=ORIENTED_EDGE('',*,*,#8792,.F.);
#12208=ORIENTED_EDGE('',*,*,#8849,.T.);
#12209=ORIENTED_EDGE('',*,*,#8683,.T.);
#12210=ORIENTED_EDGE('',*,*,#8849,.F.);
#12211=ORIENTED_EDGE('',*,*,#8791,.F.);
#12212=ORIENTED_EDGE('',*,*,#8850,.F.);
#12213=ORIENTED_EDGE('',*,*,#8684,.F.);
#12214=ORIENTED_EDGE('',*,*,#8850,.T.);
#12215=ORIENTED_EDGE('',*,*,#8790,.F.);
#12216=ORIENTED_EDGE('',*,*,#8851,.T.);
#12217=ORIENTED_EDGE('',*,*,#8685,.T.);
#12218=ORIENTED_EDGE('',*,*,#8851,.F.);
#12219=ORIENTED_EDGE('',*,*,#8789,.F.);
#12220=ORIENTED_EDGE('',*,*,#8852,.F.);
#12221=ORIENTED_EDGE('',*,*,#8686,.F.);
#12222=ORIENTED_EDGE('',*,*,#8852,.T.);
#12223=ORIENTED_EDGE('',*,*,#8788,.F.);
#12224=ORIENTED_EDGE('',*,*,#8853,.T.);
#12225=ORIENTED_EDGE('',*,*,#8687,.T.);
#12226=ORIENTED_EDGE('',*,*,#8853,.F.);
#12227=ORIENTED_EDGE('',*,*,#8787,.F.);
#12228=ORIENTED_EDGE('',*,*,#8854,.F.);
#12229=ORIENTED_EDGE('',*,*,#8688,.F.);
#12230=ORIENTED_EDGE('',*,*,#8854,.T.);
#12231=ORIENTED_EDGE('',*,*,#8786,.F.);
#12232=ORIENTED_EDGE('',*,*,#8855,.T.);
#12233=ORIENTED_EDGE('',*,*,#8689,.T.);
#12234=ORIENTED_EDGE('',*,*,#8855,.F.);
#12235=ORIENTED_EDGE('',*,*,#8785,.F.);
#12236=ORIENTED_EDGE('',*,*,#8856,.F.);
#12237=ORIENTED_EDGE('',*,*,#8690,.F.);
#12238=ORIENTED_EDGE('',*,*,#8856,.T.);
#12239=ORIENTED_EDGE('',*,*,#8784,.F.);
#12240=ORIENTED_EDGE('',*,*,#8857,.T.);
#12241=ORIENTED_EDGE('',*,*,#8691,.T.);
#12242=ORIENTED_EDGE('',*,*,#8857,.F.);
#12243=ORIENTED_EDGE('',*,*,#8783,.F.);
#12244=ORIENTED_EDGE('',*,*,#8858,.F.);
#12245=ORIENTED_EDGE('',*,*,#8692,.F.);
#12246=ORIENTED_EDGE('',*,*,#8858,.T.);
#12247=ORIENTED_EDGE('',*,*,#8782,.F.);
#12248=ORIENTED_EDGE('',*,*,#8859,.T.);
#12249=ORIENTED_EDGE('',*,*,#8693,.T.);
#12250=ORIENTED_EDGE('',*,*,#8859,.F.);
#12251=ORIENTED_EDGE('',*,*,#8781,.F.);
#12252=ORIENTED_EDGE('',*,*,#8860,.F.);
#12253=ORIENTED_EDGE('',*,*,#8694,.F.);
#12254=ORIENTED_EDGE('',*,*,#8860,.T.);
#12255=ORIENTED_EDGE('',*,*,#8780,.F.);
#12256=ORIENTED_EDGE('',*,*,#8861,.T.);
#12257=ORIENTED_EDGE('',*,*,#8695,.T.);
#12258=ORIENTED_EDGE('',*,*,#8861,.F.);
#12259=ORIENTED_EDGE('',*,*,#8779,.F.);
#12260=ORIENTED_EDGE('',*,*,#8862,.F.);
#12261=ORIENTED_EDGE('',*,*,#8696,.F.);
#12262=ORIENTED_EDGE('',*,*,#8862,.T.);
#12263=ORIENTED_EDGE('',*,*,#8778,.F.);
#12264=ORIENTED_EDGE('',*,*,#8863,.T.);
#12265=ORIENTED_EDGE('',*,*,#8697,.T.);
#12266=ORIENTED_EDGE('',*,*,#8863,.F.);
#12267=ORIENTED_EDGE('',*,*,#8777,.F.);
#12268=ORIENTED_EDGE('',*,*,#8864,.F.);
#12269=ORIENTED_EDGE('',*,*,#8698,.F.);
#12270=ORIENTED_EDGE('',*,*,#8864,.T.);
#12271=ORIENTED_EDGE('',*,*,#8776,.F.);
#12272=ORIENTED_EDGE('',*,*,#8865,.T.);
#12273=ORIENTED_EDGE('',*,*,#8699,.T.);
#12274=ORIENTED_EDGE('',*,*,#8865,.F.);
#12275=ORIENTED_EDGE('',*,*,#8775,.F.);
#12276=ORIENTED_EDGE('',*,*,#8866,.F.);
#12277=ORIENTED_EDGE('',*,*,#8700,.F.);
#12278=ORIENTED_EDGE('',*,*,#8866,.T.);
#12279=ORIENTED_EDGE('',*,*,#8774,.F.);
#12280=ORIENTED_EDGE('',*,*,#8867,.T.);
#12281=ORIENTED_EDGE('',*,*,#8701,.T.);
#12282=ORIENTED_EDGE('',*,*,#8867,.F.);
#12283=ORIENTED_EDGE('',*,*,#8773,.F.);
#12284=ORIENTED_EDGE('',*,*,#8868,.F.);
#12285=ORIENTED_EDGE('',*,*,#8702,.F.);
#12286=ORIENTED_EDGE('',*,*,#8868,.T.);
#12287=ORIENTED_EDGE('',*,*,#8772,.F.);
#12288=ORIENTED_EDGE('',*,*,#8869,.T.);
#12289=ORIENTED_EDGE('',*,*,#8703,.T.);
#12290=ORIENTED_EDGE('',*,*,#8869,.F.);
#12291=ORIENTED_EDGE('',*,*,#8771,.F.);
#12292=ORIENTED_EDGE('',*,*,#8870,.F.);
#12293=ORIENTED_EDGE('',*,*,#8704,.F.);
#12294=ORIENTED_EDGE('',*,*,#8870,.T.);
#12295=ORIENTED_EDGE('',*,*,#8770,.F.);
#12296=ORIENTED_EDGE('',*,*,#8871,.T.);
#12297=ORIENTED_EDGE('',*,*,#8705,.T.);
#12298=ORIENTED_EDGE('',*,*,#8871,.F.);
#12299=ORIENTED_EDGE('',*,*,#8769,.F.);
#12300=ORIENTED_EDGE('',*,*,#8872,.F.);
#12301=ORIENTED_EDGE('',*,*,#8706,.F.);
#12302=ORIENTED_EDGE('',*,*,#8872,.T.);
#12303=ORIENTED_EDGE('',*,*,#8768,.F.);
#12304=ORIENTED_EDGE('',*,*,#8873,.T.);
#12305=ORIENTED_EDGE('',*,*,#8707,.T.);
#12306=ORIENTED_EDGE('',*,*,#8873,.F.);
#12307=ORIENTED_EDGE('',*,*,#8767,.F.);
#12308=ORIENTED_EDGE('',*,*,#8874,.F.);
#12309=ORIENTED_EDGE('',*,*,#8708,.F.);
#12310=ORIENTED_EDGE('',*,*,#8874,.T.);
#12311=ORIENTED_EDGE('',*,*,#8766,.F.);
#12312=ORIENTED_EDGE('',*,*,#8875,.T.);
#12313=ORIENTED_EDGE('',*,*,#8709,.T.);
#12314=ORIENTED_EDGE('',*,*,#8875,.F.);
#12315=ORIENTED_EDGE('',*,*,#8765,.F.);
#12316=ORIENTED_EDGE('',*,*,#8876,.F.);
#12317=ORIENTED_EDGE('',*,*,#8710,.F.);
#12318=ORIENTED_EDGE('',*,*,#8876,.T.);
#12319=ORIENTED_EDGE('',*,*,#8764,.F.);
#12320=ORIENTED_EDGE('',*,*,#8877,.T.);
#12321=ORIENTED_EDGE('',*,*,#8711,.T.);
#12322=ORIENTED_EDGE('',*,*,#8877,.F.);
#12323=ORIENTED_EDGE('',*,*,#8763,.F.);
#12324=ORIENTED_EDGE('',*,*,#8878,.F.);
#12325=ORIENTED_EDGE('',*,*,#8712,.F.);
#12326=ORIENTED_EDGE('',*,*,#8878,.T.);
#12327=ORIENTED_EDGE('',*,*,#8762,.F.);
#12328=ORIENTED_EDGE('',*,*,#8879,.T.);
#12329=ORIENTED_EDGE('',*,*,#8713,.T.);
#12330=ORIENTED_EDGE('',*,*,#8879,.F.);
#12331=ORIENTED_EDGE('',*,*,#8761,.F.);
#12332=ORIENTED_EDGE('',*,*,#8880,.F.);
#12333=ORIENTED_EDGE('',*,*,#8714,.F.);
#12334=ORIENTED_EDGE('',*,*,#8880,.T.);
#12335=ORIENTED_EDGE('',*,*,#8760,.F.);
#12336=ORIENTED_EDGE('',*,*,#8881,.T.);
#12337=ORIENTED_EDGE('',*,*,#8715,.T.);
#12338=ORIENTED_EDGE('',*,*,#8881,.F.);
#12339=ORIENTED_EDGE('',*,*,#8759,.F.);
#12340=ORIENTED_EDGE('',*,*,#8882,.F.);
#12341=ORIENTED_EDGE('',*,*,#8716,.F.);
#12342=ORIENTED_EDGE('',*,*,#8882,.T.);
#12343=ORIENTED_EDGE('',*,*,#8758,.F.);
#12344=ORIENTED_EDGE('',*,*,#8883,.T.);
#12345=ORIENTED_EDGE('',*,*,#8717,.T.);
#12346=ORIENTED_EDGE('',*,*,#8883,.F.);
#12347=ORIENTED_EDGE('',*,*,#8757,.F.);
#12348=ORIENTED_EDGE('',*,*,#8884,.F.);
#12349=ORIENTED_EDGE('',*,*,#8718,.F.);
#12350=ORIENTED_EDGE('',*,*,#8884,.T.);
#12351=ORIENTED_EDGE('',*,*,#8756,.F.);
#12352=ORIENTED_EDGE('',*,*,#8885,.T.);
#12353=ORIENTED_EDGE('',*,*,#8719,.T.);
#12354=ORIENTED_EDGE('',*,*,#8885,.F.);
#12355=ORIENTED_EDGE('',*,*,#8755,.F.);
#12356=ORIENTED_EDGE('',*,*,#8886,.F.);
#12357=ORIENTED_EDGE('',*,*,#8720,.F.);
#12358=ORIENTED_EDGE('',*,*,#8886,.T.);
#12359=ORIENTED_EDGE('',*,*,#8754,.F.);
#12360=ORIENTED_EDGE('',*,*,#8887,.T.);
#12361=ORIENTED_EDGE('',*,*,#8721,.T.);
#12362=ORIENTED_EDGE('',*,*,#8887,.F.);
#12363=ORIENTED_EDGE('',*,*,#8753,.F.);
#12364=ORIENTED_EDGE('',*,*,#8888,.F.);
#12365=ORIENTED_EDGE('',*,*,#8722,.F.);
#12366=ORIENTED_EDGE('',*,*,#8888,.T.);
#12367=ORIENTED_EDGE('',*,*,#8752,.F.);
#12368=ORIENTED_EDGE('',*,*,#8889,.T.);
#12369=ORIENTED_EDGE('',*,*,#8723,.T.);
#12370=ORIENTED_EDGE('',*,*,#8889,.F.);
#12371=ORIENTED_EDGE('',*,*,#8751,.F.);
#12372=ORIENTED_EDGE('',*,*,#8890,.F.);
#12373=ORIENTED_EDGE('',*,*,#8724,.F.);
#12374=ORIENTED_EDGE('',*,*,#8890,.T.);
#12375=ORIENTED_EDGE('',*,*,#8750,.F.);
#12376=ORIENTED_EDGE('',*,*,#8891,.T.);
#12377=ORIENTED_EDGE('',*,*,#8725,.T.);
#12378=ORIENTED_EDGE('',*,*,#8891,.F.);
#12379=ORIENTED_EDGE('',*,*,#8749,.F.);
#12380=ORIENTED_EDGE('',*,*,#8892,.F.);
#12381=ORIENTED_EDGE('',*,*,#8726,.F.);
#12382=ORIENTED_EDGE('',*,*,#8892,.T.);
#12383=ORIENTED_EDGE('',*,*,#8748,.F.);
#12384=ORIENTED_EDGE('',*,*,#8893,.T.);
#12385=ORIENTED_EDGE('',*,*,#8727,.T.);
#12386=ORIENTED_EDGE('',*,*,#8893,.F.);
#12387=ORIENTED_EDGE('',*,*,#8747,.F.);
#12388=ORIENTED_EDGE('',*,*,#8894,.F.);
#12389=ORIENTED_EDGE('',*,*,#8728,.F.);
#12390=ORIENTED_EDGE('',*,*,#8894,.T.);
#12391=ORIENTED_EDGE('',*,*,#8746,.F.);
#12392=ORIENTED_EDGE('',*,*,#8895,.T.);
#12393=ORIENTED_EDGE('',*,*,#8729,.T.);
#12394=ORIENTED_EDGE('',*,*,#8895,.F.);
#12395=ORIENTED_EDGE('',*,*,#8745,.F.);
#12396=ORIENTED_EDGE('',*,*,#8896,.F.);
#12397=ORIENTED_EDGE('',*,*,#8730,.F.);
#12398=ORIENTED_EDGE('',*,*,#8896,.T.);
#12399=ORIENTED_EDGE('',*,*,#8744,.F.);
#12400=ORIENTED_EDGE('',*,*,#8897,.T.);
#12401=ORIENTED_EDGE('',*,*,#8731,.T.);
#12402=ORIENTED_EDGE('',*,*,#8898,.F.);
#12403=ORIENTED_EDGE('',*,*,#8732,.F.);
#12404=ORIENTED_EDGE('',*,*,#8897,.F.);
#12405=ORIENTED_EDGE('',*,*,#8743,.F.);
#12406=ORIENTED_EDGE('',*,*,#8821,.T.);
#12407=ORIENTED_EDGE('',*,*,#8735,.T.);
#12408=ORIENTED_EDGE('',*,*,#8899,.T.);
#12409=ORIENTED_EDGE('',*,*,#8740,.F.);
#12410=ORIENTED_EDGE('',*,*,#8900,.F.);
#12411=ORIENTED_EDGE('',*,*,#8741,.F.);
#12412=ORIENTED_EDGE('',*,*,#8899,.F.);
#12413=ORIENTED_EDGE('',*,*,#8734,.F.);
#12414=ORIENTED_EDGE('',*,*,#8898,.T.);
#12415=ORIENTED_EDGE('',*,*,#8742,.F.);
#12416=ORIENTED_EDGE('',*,*,#8900,.T.);
#12417=ORIENTED_EDGE('',*,*,#8733,.T.);
#12821=CYLINDRICAL_SURFACE('',#16017,0.125);
#12822=CYLINDRICAL_SURFACE('',#16018,0.125);
#12823=CYLINDRICAL_SURFACE('',#16019,1.);
#12824=CYLINDRICAL_SURFACE('',#16022,0.125);
#12825=CYLINDRICAL_SURFACE('',#16023,0.125);
#12826=CYLINDRICAL_SURFACE('',#16024,0.6);
#12827=CYLINDRICAL_SURFACE('',#16110,1.4);
#12828=CYLINDRICAL_SURFACE('',#16195,1.4);
#12829=CYLINDRICAL_SURFACE('',#16198,0.0555000000000001);
#12830=CYLINDRICAL_SURFACE('',#16199,1.24783954473516);
#12831=CYLINDRICAL_SURFACE('',#16200,0.0555000000000001);
#12832=CYLINDRICAL_SURFACE('',#16201,1.24783954473516);
#12833=CYLINDRICAL_SURFACE('',#16202,0.0555000000000001);
#12834=CYLINDRICAL_SURFACE('',#16203,1.24783954473516);
#12835=CYLINDRICAL_SURFACE('',#16204,0.0555000000000001);
#12836=CYLINDRICAL_SURFACE('',#16205,1.24783954473516);
#12837=CYLINDRICAL_SURFACE('',#16206,0.0555000000000001);
#12838=CYLINDRICAL_SURFACE('',#16207,1.24783954473516);
#12839=CYLINDRICAL_SURFACE('',#16208,0.0555000000000001);
#12840=CYLINDRICAL_SURFACE('',#16209,1.24783954473516);
#12841=CYLINDRICAL_SURFACE('',#16210,0.0555000000000001);
#12842=CYLINDRICAL_SURFACE('',#16211,1.24783954473516);
#12843=CYLINDRICAL_SURFACE('',#16212,0.0555000000000001);
#12844=CYLINDRICAL_SURFACE('',#16213,1.24783954473516);
#12845=CYLINDRICAL_SURFACE('',#16214,0.0555000000000001);
#12846=CYLINDRICAL_SURFACE('',#16215,1.24783954473516);
#12847=CYLINDRICAL_SURFACE('',#16216,0.0555000000000001);
#12848=CYLINDRICAL_SURFACE('',#16217,1.24783954473516);
#12849=CYLINDRICAL_SURFACE('',#16218,0.0555000000000001);
#12850=CYLINDRICAL_SURFACE('',#16219,1.24783954473516);
#12851=CYLINDRICAL_SURFACE('',#16220,0.0555000000000001);
#12852=CYLINDRICAL_SURFACE('',#16221,1.24783954473516);
#12853=CYLINDRICAL_SURFACE('',#16222,0.0555000000000001);
#12854=CYLINDRICAL_SURFACE('',#16223,1.24783954473516);
#12855=CYLINDRICAL_SURFACE('',#16224,0.0555000000000001);
#12856=CYLINDRICAL_SURFACE('',#16225,1.24783954473516);
#12857=CYLINDRICAL_SURFACE('',#16226,0.0555000000000001);
#12858=CYLINDRICAL_SURFACE('',#16227,1.24783954473516);
#12859=CYLINDRICAL_SURFACE('',#16228,0.0555000000000001);
#12860=CYLINDRICAL_SURFACE('',#16229,1.24783954473516);
#12861=CYLINDRICAL_SURFACE('',#16230,0.0555000000000001);
#12862=CYLINDRICAL_SURFACE('',#16231,1.24783954473516);
#12863=CYLINDRICAL_SURFACE('',#16232,0.0555000000000001);
#12864=CYLINDRICAL_SURFACE('',#16233,1.24783954473516);
#12865=CYLINDRICAL_SURFACE('',#16234,0.0555000000000001);
#12866=CYLINDRICAL_SURFACE('',#16235,1.24783954473516);
#12867=CYLINDRICAL_SURFACE('',#16236,0.0555000000000001);
#12868=CYLINDRICAL_SURFACE('',#16237,1.24783954473516);
#12869=CYLINDRICAL_SURFACE('',#16238,0.0555000000000001);
#12870=CYLINDRICAL_SURFACE('',#16239,1.24783954473516);
#12871=CYLINDRICAL_SURFACE('',#16240,0.0555000000000001);
#12872=CYLINDRICAL_SURFACE('',#16241,1.24783954473516);
#12873=CYLINDRICAL_SURFACE('',#16242,0.0555000000000001);
#12874=CYLINDRICAL_SURFACE('',#16243,1.24783954473516);
#12875=CYLINDRICAL_SURFACE('',#16244,0.0555000000000001);
#12876=CYLINDRICAL_SURFACE('',#16245,1.24783954473516);
#12877=CYLINDRICAL_SURFACE('',#16246,0.0555000000000001);
#12878=CYLINDRICAL_SURFACE('',#16247,1.24783954473516);
#12879=CYLINDRICAL_SURFACE('',#16248,0.0555000000000001);
#12880=CYLINDRICAL_SURFACE('',#16249,1.24783954473516);
#12881=CYLINDRICAL_SURFACE('',#16250,0.0555000000000001);
#12882=CYLINDRICAL_SURFACE('',#16251,1.24783954473516);
#12883=CYLINDRICAL_SURFACE('',#16252,0.0555000000000001);
#12884=CYLINDRICAL_SURFACE('',#16253,1.24783954473516);
#12885=CYLINDRICAL_SURFACE('',#16254,0.0555000000000001);
#12886=CYLINDRICAL_SURFACE('',#16255,1.24783954473516);
#12887=CYLINDRICAL_SURFACE('',#16256,0.0555000000000001);
#12888=CYLINDRICAL_SURFACE('',#16257,1.24783954473516);
#12889=CYLINDRICAL_SURFACE('',#16258,0.0555000000000001);
#12890=CYLINDRICAL_SURFACE('',#16259,1.24783954473516);
#12891=CYLINDRICAL_SURFACE('',#16260,0.0555000000000001);
#12892=CYLINDRICAL_SURFACE('',#16261,1.24783954473516);
#12893=CYLINDRICAL_SURFACE('',#16262,0.0555000000000001);
#12894=CYLINDRICAL_SURFACE('',#16263,1.24783954473516);
#12895=CYLINDRICAL_SURFACE('',#16264,0.0555000000000001);
#12896=CYLINDRICAL_SURFACE('',#16265,1.24783954473516);
#12897=CYLINDRICAL_SURFACE('',#16266,0.0555000000000001);
#12898=CYLINDRICAL_SURFACE('',#16267,1.24783954473516);
#12899=CYLINDRICAL_SURFACE('',#16268,0.0555000000000001);
#12900=CYLINDRICAL_SURFACE('',#16269,1.24783954473516);
#12901=CYLINDRICAL_SURFACE('',#16270,0.0555000000000001);
#12902=CYLINDRICAL_SURFACE('',#16271,1.24783954473516);
#12903=CYLINDRICAL_SURFACE('',#16272,0.0555000000000001);
#12904=CYLINDRICAL_SURFACE('',#16273,1.24783954473516);
#12905=CYLINDRICAL_SURFACE('',#16274,0.0555000000000001);
#12906=CYLINDRICAL_SURFACE('',#16275,1.24783954473516);
#12907=CYLINDRICAL_SURFACE('',#16276,0.0555000000000001);
#12908=CYLINDRICAL_SURFACE('',#16277,1.24783954473516);
#13590=ADVANCED_FACE('',(#2311),#12821,.F.);
#13591=ADVANCED_FACE('',(#2312),#12822,.F.);
#13592=ADVANCED_FACE('',(#2313,#1264,#1265,#1266),#12823,.T.);
#13593=ADVANCED_FACE('',(#2314),#12824,.F.);
#13594=ADVANCED_FACE('',(#2315),#12825,.F.);
#13595=ADVANCED_FACE('',(#2316,#1267,#1268,#1269),#12826,.F.);
#13596=ADVANCED_FACE('',(#2317,#1270),#1608,.F.);
#13597=ADVANCED_FACE('',(#2318,#1271),#1609,.T.);
#13598=ADVANCED_FACE('',(#2319),#12827,.T.);
#13599=ADVANCED_FACE('',(#2320,#1272),#1610,.F.);
#13600=ADVANCED_FACE('',(#2321,#1273),#1611,.F.);
#13601=ADVANCED_FACE('',(#2322),#12828,.T.);
#13602=ADVANCED_FACE('',(#2323,#1274),#1612,.T.);
#13603=ADVANCED_FACE('',(#2324),#12829,.F.);
#13604=ADVANCED_FACE('',(#2325),#12830,.T.);
#13605=ADVANCED_FACE('',(#2326),#12831,.F.);
#13606=ADVANCED_FACE('',(#2327),#12832,.T.);
#13607=ADVANCED_FACE('',(#2328),#12833,.F.);
#13608=ADVANCED_FACE('',(#2329),#12834,.T.);
#13609=ADVANCED_FACE('',(#2330),#12835,.F.);
#13610=ADVANCED_FACE('',(#2331),#12836,.T.);
#13611=ADVANCED_FACE('',(#2332),#12837,.F.);
#13612=ADVANCED_FACE('',(#2333),#12838,.T.);
#13613=ADVANCED_FACE('',(#2334),#12839,.F.);
#13614=ADVANCED_FACE('',(#2335),#12840,.T.);
#13615=ADVANCED_FACE('',(#2336),#12841,.F.);
#13616=ADVANCED_FACE('',(#2337),#12842,.T.);
#13617=ADVANCED_FACE('',(#2338),#12843,.F.);
#13618=ADVANCED_FACE('',(#2339),#12844,.T.);
#13619=ADVANCED_FACE('',(#2340),#12845,.F.);
#13620=ADVANCED_FACE('',(#2341),#12846,.T.);
#13621=ADVANCED_FACE('',(#2342),#12847,.F.);
#13622=ADVANCED_FACE('',(#2343),#12848,.T.);
#13623=ADVANCED_FACE('',(#2344),#12849,.F.);
#13624=ADVANCED_FACE('',(#2345),#12850,.T.);
#13625=ADVANCED_FACE('',(#2346),#12851,.F.);
#13626=ADVANCED_FACE('',(#2347),#12852,.T.);
#13627=ADVANCED_FACE('',(#2348),#12853,.F.);
#13628=ADVANCED_FACE('',(#2349),#12854,.T.);
#13629=ADVANCED_FACE('',(#2350),#12855,.F.);
#13630=ADVANCED_FACE('',(#2351),#12856,.T.);
#13631=ADVANCED_FACE('',(#2352),#12857,.F.);
#13632=ADVANCED_FACE('',(#2353),#12858,.T.);
#13633=ADVANCED_FACE('',(#2354),#12859,.F.);
#13634=ADVANCED_FACE('',(#2355),#12860,.T.);
#13635=ADVANCED_FACE('',(#2356),#12861,.F.);
#13636=ADVANCED_FACE('',(#2357),#12862,.T.);
#13637=ADVANCED_FACE('',(#2358),#12863,.F.);
#13638=ADVANCED_FACE('',(#2359),#12864,.T.);
#13639=ADVANCED_FACE('',(#2360),#12865,.F.);
#13640=ADVANCED_FACE('',(#2361),#12866,.T.);
#13641=ADVANCED_FACE('',(#2362),#12867,.F.);
#13642=ADVANCED_FACE('',(#2363),#12868,.T.);
#13643=ADVANCED_FACE('',(#2364),#12869,.F.);
#13644=ADVANCED_FACE('',(#2365),#12870,.T.);
#13645=ADVANCED_FACE('',(#2366),#12871,.F.);
#13646=ADVANCED_FACE('',(#2367),#12872,.T.);
#13647=ADVANCED_FACE('',(#2368),#12873,.F.);
#13648=ADVANCED_FACE('',(#2369),#12874,.T.);
#13649=ADVANCED_FACE('',(#2370),#12875,.F.);
#13650=ADVANCED_FACE('',(#2371),#12876,.T.);
#13651=ADVANCED_FACE('',(#2372),#12877,.F.);
#13652=ADVANCED_FACE('',(#2373),#12878,.T.);
#13653=ADVANCED_FACE('',(#2374),#12879,.F.);
#13654=ADVANCED_FACE('',(#2375),#12880,.T.);
#13655=ADVANCED_FACE('',(#2376),#12881,.F.);
#13656=ADVANCED_FACE('',(#2377),#12882,.T.);
#13657=ADVANCED_FACE('',(#2378),#12883,.F.);
#13658=ADVANCED_FACE('',(#2379),#12884,.T.);
#13659=ADVANCED_FACE('',(#2380),#12885,.F.);
#13660=ADVANCED_FACE('',(#2381),#12886,.T.);
#13661=ADVANCED_FACE('',(#2382),#12887,.F.);
#13662=ADVANCED_FACE('',(#2383),#12888,.T.);
#13663=ADVANCED_FACE('',(#2384),#12889,.F.);
#13664=ADVANCED_FACE('',(#2385),#12890,.T.);
#13665=ADVANCED_FACE('',(#2386),#12891,.F.);
#13666=ADVANCED_FACE('',(#2387),#12892,.T.);
#13667=ADVANCED_FACE('',(#2388),#12893,.F.);
#13668=ADVANCED_FACE('',(#2389),#12894,.T.);
#13669=ADVANCED_FACE('',(#2390),#12895,.F.);
#13670=ADVANCED_FACE('',(#2391),#12896,.T.);
#13671=ADVANCED_FACE('',(#2392),#12897,.F.);
#13672=ADVANCED_FACE('',(#2393),#12898,.T.);
#13673=ADVANCED_FACE('',(#2394),#12899,.F.);
#13674=ADVANCED_FACE('',(#2395),#12900,.T.);
#13675=ADVANCED_FACE('',(#2396),#12901,.F.);
#13676=ADVANCED_FACE('',(#2397),#12902,.T.);
#13677=ADVANCED_FACE('',(#2398),#12903,.F.);
#13678=ADVANCED_FACE('',(#2399),#12904,.T.);
#13679=ADVANCED_FACE('',(#2400),#12905,.F.);
#13680=ADVANCED_FACE('',(#2401),#12906,.T.);
#13681=ADVANCED_FACE('',(#2402),#12907,.F.);
#13682=ADVANCED_FACE('',(#2403),#12908,.T.);
#13798=CLOSED_SHELL('',(#13590,#13591,#13592,#13593,#13594,#13595,#13596,
#13597,#13598,#13599,#13600,#13601,#13602,#13603,#13604,#13605,#13606,#13607,
#13608,#13609,#13610,#13611,#13612,#13613,#13614,#13615,#13616,#13617,#13618,
#13619,#13620,#13621,#13622,#13623,#13624,#13625,#13626,#13627,#13628,#13629,
#13630,#13631,#13632,#13633,#13634,#13635,#13636,#13637,#13638,#13639,#13640,
#13641,#13642,#13643,#13644,#13645,#13646,#13647,#13648,#13649,#13650,#13651,
#13652,#13653,#13654,#13655,#13656,#13657,#13658,#13659,#13660,#13661,#13662,
#13663,#13664,#13665,#13666,#13667,#13668,#13669,#13670,#13671,#13672,#13673,
#13674,#13675,#13676,#13677,#13678,#13679,#13680,#13681,#13682));
#16016=AXIS2_PLACEMENT_3D('',#25837,#19999,#20000);
#16017=AXIS2_PLACEMENT_3D('',#25838,#20001,#20002);
#16018=AXIS2_PLACEMENT_3D('',#25925,#20004,#20005);
#16019=AXIS2_PLACEMENT_3D('',#26006,#20007,#20008);
#16020=AXIS2_PLACEMENT_3D('',#26008,#20009,#20010);
#16021=AXIS2_PLACEMENT_3D('',#26012,#20013,#20014);
#16022=AXIS2_PLACEMENT_3D('',#26095,#20015,#20016);
#16023=AXIS2_PLACEMENT_3D('',#26135,#20018,#20019);
#16024=AXIS2_PLACEMENT_3D('',#26175,#20021,#20022);
#16025=AXIS2_PLACEMENT_3D('',#26177,#20023,#20024);
#16026=AXIS2_PLACEMENT_3D('',#26181,#20027,#20028);
#16027=AXIS2_PLACEMENT_3D('',#26182,#20029,#20030);
#16028=AXIS2_PLACEMENT_3D('',#26183,#20031,#20032);
#16029=AXIS2_PLACEMENT_3D('',#26185,#20033,#20034);
#16030=AXIS2_PLACEMENT_3D('',#26188,#20035,#20036);
#16031=AXIS2_PLACEMENT_3D('',#26190,#20037,#20038);
#16032=AXIS2_PLACEMENT_3D('',#26192,#20039,#20040);
#16033=AXIS2_PLACEMENT_3D('',#26194,#20041,#20042);
#16034=AXIS2_PLACEMENT_3D('',#26196,#20043,#20044);
#16035=AXIS2_PLACEMENT_3D('',#26198,#20045,#20046);
#16036=AXIS2_PLACEMENT_3D('',#26200,#20047,#20048);
#16037=AXIS2_PLACEMENT_3D('',#26202,#20049,#20050);
#16038=AXIS2_PLACEMENT_3D('',#26204,#20051,#20052);
#16039=AXIS2_PLACEMENT_3D('',#26206,#20053,#20054);
#16040=AXIS2_PLACEMENT_3D('',#26208,#20055,#20056);
#16041=AXIS2_PLACEMENT_3D('',#26210,#20057,#20058);
#16042=AXIS2_PLACEMENT_3D('',#26212,#20059,#20060);
#16043=AXIS2_PLACEMENT_3D('',#26214,#20061,#20062);
#16044=AXIS2_PLACEMENT_3D('',#26216,#20063,#20064);
#16045=AXIS2_PLACEMENT_3D('',#26218,#20065,#20066);
#16046=AXIS2_PLACEMENT_3D('',#26220,#20067,#20068);
#16047=AXIS2_PLACEMENT_3D('',#26222,#20069,#20070);
#16048=AXIS2_PLACEMENT_3D('',#26224,#20071,#20072);
#16049=AXIS2_PLACEMENT_3D('',#26226,#20073,#20074);
#16050=AXIS2_PLACEMENT_3D('',#26228,#20075,#20076);
#16051=AXIS2_PLACEMENT_3D('',#26230,#20077,#20078);
#16052=AXIS2_PLACEMENT_3D('',#26232,#20079,#20080);
#16053=AXIS2_PLACEMENT_3D('',#26234,#20081,#20082);
#16054=AXIS2_PLACEMENT_3D('',#26236,#20083,#20084);
#16055=AXIS2_PLACEMENT_3D('',#26238,#20085,#20086);
#16056=AXIS2_PLACEMENT_3D('',#26240,#20087,#20088);
#16057=AXIS2_PLACEMENT_3D('',#26242,#20089,#20090);
#16058=AXIS2_PLACEMENT_3D('',#26244,#20091,#20092);
#16059=AXIS2_PLACEMENT_3D('',#26246,#20093,#20094);
#16060=AXIS2_PLACEMENT_3D('',#26248,#20095,#20096);
#16061=AXIS2_PLACEMENT_3D('',#26250,#20097,#20098);
#16062=AXIS2_PLACEMENT_3D('',#26252,#20099,#20100);
#16063=AXIS2_PLACEMENT_3D('',#26254,#20101,#20102);
#16064=AXIS2_PLACEMENT_3D('',#26256,#20103,#20104);
#16065=AXIS2_PLACEMENT_3D('',#26258,#20105,#20106);
#16066=AXIS2_PLACEMENT_3D('',#26260,#20107,#20108);
#16067=AXIS2_PLACEMENT_3D('',#26262,#20109,#20110);
#16068=AXIS2_PLACEMENT_3D('',#26264,#20111,#20112);
#16069=AXIS2_PLACEMENT_3D('',#26266,#20113,#20114);
#16070=AXIS2_PLACEMENT_3D('',#26268,#20115,#20116);
#16071=AXIS2_PLACEMENT_3D('',#26270,#20117,#20118);
#16072=AXIS2_PLACEMENT_3D('',#26272,#20119,#20120);
#16073=AXIS2_PLACEMENT_3D('',#26274,#20121,#20122);
#16074=AXIS2_PLACEMENT_3D('',#26276,#20123,#20124);
#16075=AXIS2_PLACEMENT_3D('',#26278,#20125,#20126);
#16076=AXIS2_PLACEMENT_3D('',#26280,#20127,#20128);
#16077=AXIS2_PLACEMENT_3D('',#26282,#20129,#20130);
#16078=AXIS2_PLACEMENT_3D('',#26284,#20131,#20132);
#16079=AXIS2_PLACEMENT_3D('',#26286,#20133,#20134);
#16080=AXIS2_PLACEMENT_3D('',#26288,#20135,#20136);
#16081=AXIS2_PLACEMENT_3D('',#26290,#20137,#20138);
#16082=AXIS2_PLACEMENT_3D('',#26292,#20139,#20140);
#16083=AXIS2_PLACEMENT_3D('',#26294,#20141,#20142);
#16084=AXIS2_PLACEMENT_3D('',#26296,#20143,#20144);
#16085=AXIS2_PLACEMENT_3D('',#26298,#20145,#20146);
#16086=AXIS2_PLACEMENT_3D('',#26300,#20147,#20148);
#16087=AXIS2_PLACEMENT_3D('',#26302,#20149,#20150);
#16088=AXIS2_PLACEMENT_3D('',#26304,#20151,#20152);
#16089=AXIS2_PLACEMENT_3D('',#26306,#20153,#20154);
#16090=AXIS2_PLACEMENT_3D('',#26308,#20155,#20156);
#16091=AXIS2_PLACEMENT_3D('',#26310,#20157,#20158);
#16092=AXIS2_PLACEMENT_3D('',#26312,#20159,#20160);
#16093=AXIS2_PLACEMENT_3D('',#26314,#20161,#20162);
#16094=AXIS2_PLACEMENT_3D('',#26316,#20163,#20164);
#16095=AXIS2_PLACEMENT_3D('',#26318,#20165,#20166);
#16096=AXIS2_PLACEMENT_3D('',#26320,#20167,#20168);
#16097=AXIS2_PLACEMENT_3D('',#26322,#20169,#20170);
#16098=AXIS2_PLACEMENT_3D('',#26324,#20171,#20172);
#16099=AXIS2_PLACEMENT_3D('',#26326,#20173,#20174);
#16100=AXIS2_PLACEMENT_3D('',#26328,#20175,#20176);
#16101=AXIS2_PLACEMENT_3D('',#26330,#20177,#20178);
#16102=AXIS2_PLACEMENT_3D('',#26332,#20179,#20180);
#16103=AXIS2_PLACEMENT_3D('',#26334,#20181,#20182);
#16104=AXIS2_PLACEMENT_3D('',#26336,#20183,#20184);
#16105=AXIS2_PLACEMENT_3D('',#26338,#20185,#20186);
#16106=AXIS2_PLACEMENT_3D('',#26340,#20187,#20188);
#16107=AXIS2_PLACEMENT_3D('',#26342,#20189,#20190);
#16108=AXIS2_PLACEMENT_3D('',#26344,#20191,#20192);
#16109=AXIS2_PLACEMENT_3D('',#26345,#20193,#20194);
#16110=AXIS2_PLACEMENT_3D('',#26346,#20195,#20196);
#16111=AXIS2_PLACEMENT_3D('',#26348,#20197,#20198);
#16112=AXIS2_PLACEMENT_3D('',#26350,#20200,#20201);
#16113=AXIS2_PLACEMENT_3D('',#26351,#20202,#20203);
#16114=AXIS2_PLACEMENT_3D('',#26353,#20204,#20205);
#16115=AXIS2_PLACEMENT_3D('',#26356,#20206,#20207);
#16116=AXIS2_PLACEMENT_3D('',#26358,#20208,#20209);
#16117=AXIS2_PLACEMENT_3D('',#26360,#20210,#20211);
#16118=AXIS2_PLACEMENT_3D('',#26362,#20212,#20213);
#16119=AXIS2_PLACEMENT_3D('',#26364,#20214,#20215);
#16120=AXIS2_PLACEMENT_3D('',#26366,#20216,#20217);
#16121=AXIS2_PLACEMENT_3D('',#26368,#20218,#20219);
#16122=AXIS2_PLACEMENT_3D('',#26370,#20220,#20221);
#16123=AXIS2_PLACEMENT_3D('',#26372,#20222,#20223);
#16124=AXIS2_PLACEMENT_3D('',#26374,#20224,#20225);
#16125=AXIS2_PLACEMENT_3D('',#26376,#20226,#20227);
#16126=AXIS2_PLACEMENT_3D('',#26378,#20228,#20229);
#16127=AXIS2_PLACEMENT_3D('',#26380,#20230,#20231);
#16128=AXIS2_PLACEMENT_3D('',#26382,#20232,#20233);
#16129=AXIS2_PLACEMENT_3D('',#26384,#20234,#20235);
#16130=AXIS2_PLACEMENT_3D('',#26386,#20236,#20237);
#16131=AXIS2_PLACEMENT_3D('',#26388,#20238,#20239);
#16132=AXIS2_PLACEMENT_3D('',#26390,#20240,#20241);
#16133=AXIS2_PLACEMENT_3D('',#26392,#20242,#20243);
#16134=AXIS2_PLACEMENT_3D('',#26394,#20244,#20245);
#16135=AXIS2_PLACEMENT_3D('',#26396,#20246,#20247);
#16136=AXIS2_PLACEMENT_3D('',#26398,#20248,#20249);
#16137=AXIS2_PLACEMENT_3D('',#26400,#20250,#20251);
#16138=AXIS2_PLACEMENT_3D('',#26402,#20252,#20253);
#16139=AXIS2_PLACEMENT_3D('',#26404,#20254,#20255);
#16140=AXIS2_PLACEMENT_3D('',#26406,#20256,#20257);
#16141=AXIS2_PLACEMENT_3D('',#26408,#20258,#20259);
#16142=AXIS2_PLACEMENT_3D('',#26410,#20260,#20261);
#16143=AXIS2_PLACEMENT_3D('',#26412,#20262,#20263);
#16144=AXIS2_PLACEMENT_3D('',#26414,#20264,#20265);
#16145=AXIS2_PLACEMENT_3D('',#26416,#20266,#20267);
#16146=AXIS2_PLACEMENT_3D('',#26418,#20268,#20269);
#16147=AXIS2_PLACEMENT_3D('',#26420,#20270,#20271);
#16148=AXIS2_PLACEMENT_3D('',#26422,#20272,#20273);
#16149=AXIS2_PLACEMENT_3D('',#26424,#20274,#20275);
#16150=AXIS2_PLACEMENT_3D('',#26426,#20276,#20277);
#16151=AXIS2_PLACEMENT_3D('',#26428,#20278,#20279);
#16152=AXIS2_PLACEMENT_3D('',#26430,#20280,#20281);
#16153=AXIS2_PLACEMENT_3D('',#26432,#20282,#20283);
#16154=AXIS2_PLACEMENT_3D('',#26434,#20284,#20285);
#16155=AXIS2_PLACEMENT_3D('',#26436,#20286,#20287);
#16156=AXIS2_PLACEMENT_3D('',#26438,#20288,#20289);
#16157=AXIS2_PLACEMENT_3D('',#26440,#20290,#20291);
#16158=AXIS2_PLACEMENT_3D('',#26442,#20292,#20293);
#16159=AXIS2_PLACEMENT_3D('',#26444,#20294,#20295);
#16160=AXIS2_PLACEMENT_3D('',#26446,#20296,#20297);
#16161=AXIS2_PLACEMENT_3D('',#26448,#20298,#20299);
#16162=AXIS2_PLACEMENT_3D('',#26450,#20300,#20301);
#16163=AXIS2_PLACEMENT_3D('',#26452,#20302,#20303);
#16164=AXIS2_PLACEMENT_3D('',#26454,#20304,#20305);
#16165=AXIS2_PLACEMENT_3D('',#26456,#20306,#20307);
#16166=AXIS2_PLACEMENT_3D('',#26458,#20308,#20309);
#16167=AXIS2_PLACEMENT_3D('',#26460,#20310,#20311);
#16168=AXIS2_PLACEMENT_3D('',#26462,#20312,#20313);
#16169=AXIS2_PLACEMENT_3D('',#26464,#20314,#20315);
#16170=AXIS2_PLACEMENT_3D('',#26466,#20316,#20317);
#16171=AXIS2_PLACEMENT_3D('',#26468,#20318,#20319);
#16172=AXIS2_PLACEMENT_3D('',#26470,#20320,#20321);
#16173=AXIS2_PLACEMENT_3D('',#26472,#20322,#20323);
#16174=AXIS2_PLACEMENT_3D('',#26474,#20324,#20325);
#16175=AXIS2_PLACEMENT_3D('',#26476,#20326,#20327);
#16176=AXIS2_PLACEMENT_3D('',#26478,#20328,#20329);
#16177=AXIS2_PLACEMENT_3D('',#26480,#20330,#20331);
#16178=AXIS2_PLACEMENT_3D('',#26482,#20332,#20333);
#16179=AXIS2_PLACEMENT_3D('',#26484,#20334,#20335);
#16180=AXIS2_PLACEMENT_3D('',#26486,#20336,#20337);
#16181=AXIS2_PLACEMENT_3D('',#26488,#20338,#20339);
#16182=AXIS2_PLACEMENT_3D('',#26490,#20340,#20341);
#16183=AXIS2_PLACEMENT_3D('',#26492,#20342,#20343);
#16184=AXIS2_PLACEMENT_3D('',#26494,#20344,#20345);
#16185=AXIS2_PLACEMENT_3D('',#26496,#20346,#20347);
#16186=AXIS2_PLACEMENT_3D('',#26498,#20348,#20349);
#16187=AXIS2_PLACEMENT_3D('',#26500,#20350,#20351);
#16188=AXIS2_PLACEMENT_3D('',#26502,#20352,#20353);
#16189=AXIS2_PLACEMENT_3D('',#26504,#20354,#20355);
#16190=AXIS2_PLACEMENT_3D('',#26506,#20356,#20357);
#16191=AXIS2_PLACEMENT_3D('',#26508,#20358,#20359);
#16192=AXIS2_PLACEMENT_3D('',#26510,#20360,#20361);
#16193=AXIS2_PLACEMENT_3D('',#26512,#20362,#20363);
#16194=AXIS2_PLACEMENT_3D('',#26513,#20364,#20365);
#16195=AXIS2_PLACEMENT_3D('',#26514,#20366,#20367);
#16196=AXIS2_PLACEMENT_3D('',#26516,#20368,#20369);
#16197=AXIS2_PLACEMENT_3D('',#26518,#20371,#20372);
#16198=AXIS2_PLACEMENT_3D('',#26519,#20373,#20374);
#16199=AXIS2_PLACEMENT_3D('',#26522,#20377,#20378);
#16200=AXIS2_PLACEMENT_3D('',#26524,#20380,#20381);
#16201=AXIS2_PLACEMENT_3D('',#26526,#20383,#20384);
#16202=AXIS2_PLACEMENT_3D('',#26528,#20386,#20387);
#16203=AXIS2_PLACEMENT_3D('',#26530,#20389,#20390);
#16204=AXIS2_PLACEMENT_3D('',#26532,#20392,#20393);
#16205=AXIS2_PLACEMENT_3D('',#26534,#20395,#20396);
#16206=AXIS2_PLACEMENT_3D('',#26536,#20398,#20399);
#16207=AXIS2_PLACEMENT_3D('',#26538,#20401,#20402);
#16208=AXIS2_PLACEMENT_3D('',#26540,#20404,#20405);
#16209=AXIS2_PLACEMENT_3D('',#26542,#20407,#20408);
#16210=AXIS2_PLACEMENT_3D('',#26544,#20410,#20411);
#16211=AXIS2_PLACEMENT_3D('',#26546,#20413,#20414);
#16212=AXIS2_PLACEMENT_3D('',#26548,#20416,#20417);
#16213=AXIS2_PLACEMENT_3D('',#26550,#20419,#20420);
#16214=AXIS2_PLACEMENT_3D('',#26552,#20422,#20423);
#16215=AXIS2_PLACEMENT_3D('',#26554,#20425,#20426);
#16216=AXIS2_PLACEMENT_3D('',#26556,#20428,#20429);
#16217=AXIS2_PLACEMENT_3D('',#26558,#20431,#20432);
#16218=AXIS2_PLACEMENT_3D('',#26560,#20434,#20435);
#16219=AXIS2_PLACEMENT_3D('',#26562,#20437,#20438);
#16220=AXIS2_PLACEMENT_3D('',#26564,#20440,#20441);
#16221=AXIS2_PLACEMENT_3D('',#26566,#20443,#20444);
#16222=AXIS2_PLACEMENT_3D('',#26568,#20446,#20447);
#16223=AXIS2_PLACEMENT_3D('',#26570,#20449,#20450);
#16224=AXIS2_PLACEMENT_3D('',#26572,#20452,#20453);
#16225=AXIS2_PLACEMENT_3D('',#26574,#20455,#20456);
#16226=AXIS2_PLACEMENT_3D('',#26576,#20458,#20459);
#16227=AXIS2_PLACEMENT_3D('',#26578,#20461,#20462);
#16228=AXIS2_PLACEMENT_3D('',#26580,#20464,#20465);
#16229=AXIS2_PLACEMENT_3D('',#26582,#20467,#20468);
#16230=AXIS2_PLACEMENT_3D('',#26584,#20470,#20471);
#16231=AXIS2_PLACEMENT_3D('',#26586,#20473,#20474);
#16232=AXIS2_PLACEMENT_3D('',#26588,#20476,#20477);
#16233=AXIS2_PLACEMENT_3D('',#26590,#20479,#20480);
#16234=AXIS2_PLACEMENT_3D('',#26592,#20482,#20483);
#16235=AXIS2_PLACEMENT_3D('',#26594,#20485,#20486);
#16236=AXIS2_PLACEMENT_3D('',#26596,#20488,#20489);
#16237=AXIS2_PLACEMENT_3D('',#26598,#20491,#20492);
#16238=AXIS2_PLACEMENT_3D('',#26600,#20494,#20495);
#16239=AXIS2_PLACEMENT_3D('',#26602,#20497,#20498);
#16240=AXIS2_PLACEMENT_3D('',#26604,#20500,#20501);
#16241=AXIS2_PLACEMENT_3D('',#26606,#20503,#20504);
#16242=AXIS2_PLACEMENT_3D('',#26608,#20506,#20507);
#16243=AXIS2_PLACEMENT_3D('',#26610,#20509,#20510);
#16244=AXIS2_PLACEMENT_3D('',#26612,#20512,#20513);
#16245=AXIS2_PLACEMENT_3D('',#26614,#20515,#20516);
#16246=AXIS2_PLACEMENT_3D('',#26616,#20518,#20519);
#16247=AXIS2_PLACEMENT_3D('',#26618,#20521,#20522);
#16248=AXIS2_PLACEMENT_3D('',#26620,#20524,#20525);
#16249=AXIS2_PLACEMENT_3D('',#26622,#20527,#20528);
#16250=AXIS2_PLACEMENT_3D('',#26624,#20530,#20531);
#16251=AXIS2_PLACEMENT_3D('',#26626,#20533,#20534);
#16252=AXIS2_PLACEMENT_3D('',#26628,#20536,#20537);
#16253=AXIS2_PLACEMENT_3D('',#26630,#20539,#20540);
#16254=AXIS2_PLACEMENT_3D('',#26632,#20542,#20543);
#16255=AXIS2_PLACEMENT_3D('',#26634,#20545,#20546);
#16256=AXIS2_PLACEMENT_3D('',#26636,#20548,#20549);
#16257=AXIS2_PLACEMENT_3D('',#26638,#20551,#20552);
#16258=AXIS2_PLACEMENT_3D('',#26640,#20554,#20555);
#16259=AXIS2_PLACEMENT_3D('',#26642,#20557,#20558);
#16260=AXIS2_PLACEMENT_3D('',#26644,#20560,#20561);
#16261=AXIS2_PLACEMENT_3D('',#26646,#20563,#20564);
#16262=AXIS2_PLACEMENT_3D('',#26648,#20566,#20567);
#16263=AXIS2_PLACEMENT_3D('',#26650,#20569,#20570);
#16264=AXIS2_PLACEMENT_3D('',#26652,#20572,#20573);
#16265=AXIS2_PLACEMENT_3D('',#26654,#20575,#20576);
#16266=AXIS2_PLACEMENT_3D('',#26656,#20578,#20579);
#16267=AXIS2_PLACEMENT_3D('',#26658,#20581,#20582);
#16268=AXIS2_PLACEMENT_3D('',#26660,#20584,#20585);
#16269=AXIS2_PLACEMENT_3D('',#26662,#20587,#20588);
#16270=AXIS2_PLACEMENT_3D('',#26664,#20590,#20591);
#16271=AXIS2_PLACEMENT_3D('',#26666,#20593,#20594);
#16272=AXIS2_PLACEMENT_3D('',#26668,#20596,#20597);
#16273=AXIS2_PLACEMENT_3D('',#26670,#20599,#20600);
#16274=AXIS2_PLACEMENT_3D('',#26672,#20602,#20603);
#16275=AXIS2_PLACEMENT_3D('',#26674,#20605,#20606);
#16276=AXIS2_PLACEMENT_3D('',#26676,#20608,#20609);
#16277=AXIS2_PLACEMENT_3D('',#26678,#20611,#20612);
#19999=DIRECTION('axis',(0.,0.,1.));
#20000=DIRECTION('refdir',(1.,0.,0.));
#20001=DIRECTION('center_axis',(1.,0.,6.12323399573677E-17));
#20002=DIRECTION('ref_axis',(6.12323399573677E-17,0.,-1.));
#20003=DIRECTION('',(1.,0.,6.12323399573677E-17));
#20004=DIRECTION('center_axis',(1.,0.,6.12323399573677E-17));
#20005=DIRECTION('ref_axis',(6.12323399573677E-17,0.,-1.));
#20006=DIRECTION('',(1.,0.,6.12323399573677E-17));
#20007=DIRECTION('center_axis',(0.,-1.,0.));
#20008=DIRECTION('ref_axis',(1.,0.,0.));
#20009=DIRECTION('center_axis',(0.,-1.,0.));
#20010=DIRECTION('ref_axis',(1.,0.,0.));
#20011=DIRECTION('',(0.,1.,0.));
#20012=DIRECTION('',(0.,1.,0.));
#20013=DIRECTION('center_axis',(0.,1.,0.));
#20014=DIRECTION('ref_axis',(1.,0.,0.));
#20015=DIRECTION('center_axis',(0.,0.,1.));
#20016=DIRECTION('ref_axis',(1.,0.,0.));
#20017=DIRECTION('',(0.,0.,1.));
#20018=DIRECTION('center_axis',(0.,0.,1.));
#20019=DIRECTION('ref_axis',(1.,0.,0.));
#20020=DIRECTION('',(0.,0.,1.));
#20021=DIRECTION('center_axis',(0.,1.,0.));
#20022=DIRECTION('ref_axis',(1.,0.,0.));
#20023=DIRECTION('center_axis',(0.,1.,0.));
#20024=DIRECTION('ref_axis',(1.,0.,0.));
#20025=DIRECTION('',(0.,1.,0.));
#20026=DIRECTION('',(0.,1.,0.));
#20027=DIRECTION('center_axis',(0.,-1.,0.));
#20028=DIRECTION('ref_axis',(1.,0.,0.));
#20029=DIRECTION('center_axis',(0.,1.,0.));
#20030=DIRECTION('ref_axis',(1.,0.,0.));
#20031=DIRECTION('center_axis',(0.,1.,0.));
#20032=DIRECTION('ref_axis',(1.,0.,0.));
#20033=DIRECTION('center_axis',(0.,1.,0.));
#20034=DIRECTION('ref_axis',(1.,0.,0.));
#20035=DIRECTION('center_axis',(0.,1.,0.));
#20036=DIRECTION('ref_axis',(0.987688340595138,0.,0.156434465040231));
#20037=DIRECTION('center_axis',(0.,1.,0.));
#20038=DIRECTION('ref_axis',(1.,0.,0.));
#20039=DIRECTION('center_axis',(0.,1.,0.));
#20040=DIRECTION('ref_axis',(0.951056516295154,0.,0.309016994374948));
#20041=DIRECTION('center_axis',(0.,1.,0.));
#20042=DIRECTION('ref_axis',(1.,0.,0.));
#20043=DIRECTION('center_axis',(0.,1.,0.));
#20044=DIRECTION('ref_axis',(0.891006524188368,0.,0.453990499739547));
#20045=DIRECTION('center_axis',(0.,1.,0.));
#20046=DIRECTION('ref_axis',(1.,0.,0.));
#20047=DIRECTION('center_axis',(0.,1.,0.));
#20048=DIRECTION('ref_axis',(0.809016994374947,0.,0.587785252292473));
#20049=DIRECTION('center_axis',(0.,1.,0.));
#20050=DIRECTION('ref_axis',(1.,0.,0.));
#20051=DIRECTION('center_axis',(0.,1.,0.));
#20052=DIRECTION('ref_axis',(0.707106781186547,0.,0.707106781186548));
#20053=DIRECTION('center_axis',(0.,1.,0.));
#20054=DIRECTION('ref_axis',(1.,0.,0.));
#20055=DIRECTION('center_axis',(0.,1.,0.));
#20056=DIRECTION('ref_axis',(0.587785252292473,0.,0.809016994374948));
#20057=DIRECTION('center_axis',(0.,1.,0.));
#20058=DIRECTION('ref_axis',(1.,0.,0.));
#20059=DIRECTION('center_axis',(0.,1.,0.));
#20060=DIRECTION('ref_axis',(0.453990499739547,0.,0.891006524188368));
#20061=DIRECTION('center_axis',(0.,1.,0.));
#20062=DIRECTION('ref_axis',(1.,0.,0.));
#20063=DIRECTION('center_axis',(0.,1.,0.));
#20064=DIRECTION('ref_axis',(0.309016994374947,0.,0.951056516295154));
#20065=DIRECTION('center_axis',(0.,1.,0.));
#20066=DIRECTION('ref_axis',(1.,0.,0.));
#20067=DIRECTION('center_axis',(0.,1.,0.));
#20068=DIRECTION('ref_axis',(0.156434465040231,0.,0.987688340595138));
#20069=DIRECTION('center_axis',(0.,1.,0.));
#20070=DIRECTION('ref_axis',(1.,0.,0.));
#20071=DIRECTION('center_axis',(0.,1.,0.));
#20072=DIRECTION('ref_axis',(-1.83697019872103E-16,0.,1.));
#20073=DIRECTION('center_axis',(0.,1.,0.));
#20074=DIRECTION('ref_axis',(1.,0.,0.));
#20075=DIRECTION('center_axis',(0.,1.,0.));
#20076=DIRECTION('ref_axis',(-0.156434465040231,0.,0.987688340595138));
#20077=DIRECTION('center_axis',(0.,1.,0.));
#20078=DIRECTION('ref_axis',(1.,0.,0.));
#20079=DIRECTION('center_axis',(0.,1.,0.));
#20080=DIRECTION('ref_axis',(-0.309016994374948,0.,0.951056516295154));
#20081=DIRECTION('center_axis',(0.,1.,0.));
#20082=DIRECTION('ref_axis',(1.,0.,0.));
#20083=DIRECTION('center_axis',(0.,1.,0.));
#20084=DIRECTION('ref_axis',(-0.453990499739547,0.,0.891006524188368));
#20085=DIRECTION('center_axis',(0.,1.,0.));
#20086=DIRECTION('ref_axis',(1.,0.,0.));
#20087=DIRECTION('center_axis',(0.,1.,0.));
#20088=DIRECTION('ref_axis',(-0.587785252292473,0.,0.809016994374947));
#20089=DIRECTION('center_axis',(0.,1.,0.));
#20090=DIRECTION('ref_axis',(1.,0.,0.));
#20091=DIRECTION('center_axis',(0.,1.,0.));
#20092=DIRECTION('ref_axis',(-0.707106781186548,0.,0.707106781186547));
#20093=DIRECTION('center_axis',(0.,1.,0.));
#20094=DIRECTION('ref_axis',(1.,0.,0.));
#20095=DIRECTION('center_axis',(0.,1.,0.));
#20096=DIRECTION('ref_axis',(-0.809016994374947,0.,0.587785252292473));
#20097=DIRECTION('center_axis',(0.,1.,0.));
#20098=DIRECTION('ref_axis',(1.,0.,0.));
#20099=DIRECTION('center_axis',(0.,1.,0.));
#20100=DIRECTION('ref_axis',(-0.891006524188368,0.,0.453990499739547));
#20101=DIRECTION('center_axis',(0.,1.,0.));
#20102=DIRECTION('ref_axis',(1.,0.,0.));
#20103=DIRECTION('center_axis',(0.,1.,0.));
#20104=DIRECTION('ref_axis',(-0.951056516295154,0.,0.309016994374947));
#20105=DIRECTION('center_axis',(0.,1.,0.));
#20106=DIRECTION('ref_axis',(1.,0.,0.));
#20107=DIRECTION('center_axis',(0.,1.,0.));
#20108=DIRECTION('ref_axis',(-0.987688340595138,0.,0.156434465040231));
#20109=DIRECTION('center_axis',(0.,1.,0.));
#20110=DIRECTION('ref_axis',(1.,0.,0.));
#20111=DIRECTION('center_axis',(0.,1.,0.));
#20112=DIRECTION('ref_axis',(-1.,0.,-1.22464679914735E-16));
#20113=DIRECTION('center_axis',(0.,1.,0.));
#20114=DIRECTION('ref_axis',(1.,0.,0.));
#20115=DIRECTION('center_axis',(0.,1.,0.));
#20116=DIRECTION('ref_axis',(-0.987688340595138,0.,-0.156434465040231));
#20117=DIRECTION('center_axis',(0.,1.,0.));
#20118=DIRECTION('ref_axis',(1.,0.,0.));
#20119=DIRECTION('center_axis',(0.,1.,0.));
#20120=DIRECTION('ref_axis',(-0.951056516295154,0.,-0.309016994374948));
#20121=DIRECTION('center_axis',(0.,1.,0.));
#20122=DIRECTION('ref_axis',(1.,0.,0.));
#20123=DIRECTION('center_axis',(0.,1.,0.));
#20124=DIRECTION('ref_axis',(-0.891006524188368,0.,-0.453990499739547));
#20125=DIRECTION('center_axis',(0.,1.,0.));
#20126=DIRECTION('ref_axis',(1.,0.,0.));
#20127=DIRECTION('center_axis',(0.,1.,0.));
#20128=DIRECTION('ref_axis',(-0.809016994374947,0.,-0.587785252292473));
#20129=DIRECTION('center_axis',(0.,1.,0.));
#20130=DIRECTION('ref_axis',(1.,0.,0.));
#20131=DIRECTION('center_axis',(0.,1.,0.));
#20132=DIRECTION('ref_axis',(-0.707106781186547,0.,-0.707106781186548));
#20133=DIRECTION('center_axis',(0.,1.,0.));
#20134=DIRECTION('ref_axis',(1.,0.,0.));
#20135=DIRECTION('center_axis',(0.,1.,0.));
#20136=DIRECTION('ref_axis',(-0.587785252292473,0.,-0.809016994374947));
#20137=DIRECTION('center_axis',(0.,1.,0.));
#20138=DIRECTION('ref_axis',(1.,0.,0.));
#20139=DIRECTION('center_axis',(0.,1.,0.));
#20140=DIRECTION('ref_axis',(-0.453990499739547,0.,-0.891006524188368));
#20141=DIRECTION('center_axis',(0.,1.,0.));
#20142=DIRECTION('ref_axis',(1.,0.,0.));
#20143=DIRECTION('center_axis',(0.,1.,0.));
#20144=DIRECTION('ref_axis',(-0.309016994374947,0.,-0.951056516295154));
#20145=DIRECTION('center_axis',(0.,1.,0.));
#20146=DIRECTION('ref_axis',(1.,0.,0.));
#20147=DIRECTION('center_axis',(0.,1.,0.));
#20148=DIRECTION('ref_axis',(-0.156434465040231,0.,-0.987688340595138));
#20149=DIRECTION('center_axis',(0.,1.,0.));
#20150=DIRECTION('ref_axis',(1.,0.,0.));
#20151=DIRECTION('center_axis',(0.,1.,0.));
#20152=DIRECTION('ref_axis',(6.12323399573677E-17,0.,-1.));
#20153=DIRECTION('center_axis',(0.,1.,0.));
#20154=DIRECTION('ref_axis',(1.,0.,0.));
#20155=DIRECTION('center_axis',(0.,1.,0.));
#20156=DIRECTION('ref_axis',(0.156434465040231,0.,-0.987688340595138));
#20157=DIRECTION('center_axis',(0.,1.,0.));
#20158=DIRECTION('ref_axis',(1.,0.,0.));
#20159=DIRECTION('center_axis',(0.,1.,0.));
#20160=DIRECTION('ref_axis',(0.309016994374948,0.,-0.951056516295154));
#20161=DIRECTION('center_axis',(0.,1.,0.));
#20162=DIRECTION('ref_axis',(1.,0.,0.));
#20163=DIRECTION('center_axis',(0.,1.,0.));
#20164=DIRECTION('ref_axis',(0.453990499739547,0.,-0.891006524188368));
#20165=DIRECTION('center_axis',(0.,1.,0.));
#20166=DIRECTION('ref_axis',(1.,0.,0.));
#20167=DIRECTION('center_axis',(0.,1.,0.));
#20168=DIRECTION('ref_axis',(0.587785252292473,0.,-0.809016994374947));
#20169=DIRECTION('center_axis',(0.,1.,0.));
#20170=DIRECTION('ref_axis',(1.,0.,0.));
#20171=DIRECTION('center_axis',(0.,1.,0.));
#20172=DIRECTION('ref_axis',(0.707106781186548,0.,-0.707106781186547));
#20173=DIRECTION('center_axis',(0.,1.,0.));
#20174=DIRECTION('ref_axis',(1.,0.,0.));
#20175=DIRECTION('center_axis',(0.,1.,0.));
#20176=DIRECTION('ref_axis',(0.809016994374947,0.,-0.587785252292473));
#20177=DIRECTION('center_axis',(0.,1.,0.));
#20178=DIRECTION('ref_axis',(1.,0.,0.));
#20179=DIRECTION('center_axis',(0.,1.,0.));
#20180=DIRECTION('ref_axis',(0.891006524188368,0.,-0.453990499739547));
#20181=DIRECTION('center_axis',(0.,1.,0.));
#20182=DIRECTION('ref_axis',(1.,0.,0.));
#20183=DIRECTION('center_axis',(0.,1.,0.));
#20184=DIRECTION('ref_axis',(0.951056516295154,0.,-0.309016994374947));
#20185=DIRECTION('center_axis',(0.,1.,0.));
#20186=DIRECTION('ref_axis',(1.,0.,0.));
#20187=DIRECTION('center_axis',(0.,1.,0.));
#20188=DIRECTION('ref_axis',(0.987688340595138,0.,-0.156434465040231));
#20189=DIRECTION('center_axis',(0.,1.,0.));
#20190=DIRECTION('ref_axis',(1.,0.,0.));
#20191=DIRECTION('center_axis',(0.,1.,0.));
#20192=DIRECTION('ref_axis',(1.,0.,0.));
#20193=DIRECTION('center_axis',(0.,1.,0.));
#20194=DIRECTION('ref_axis',(1.,0.,0.));
#20195=DIRECTION('center_axis',(0.,-1.,0.));
#20196=DIRECTION('ref_axis',(1.,0.,0.));
#20197=DIRECTION('center_axis',(0.,-1.,0.));
#20198=DIRECTION('ref_axis',(1.,0.,0.));
#20199=DIRECTION('',(0.,1.,0.));
#20200=DIRECTION('center_axis',(0.,1.,0.));
#20201=DIRECTION('ref_axis',(1.,0.,0.));
#20202=DIRECTION('center_axis',(0.,1.,0.));
#20203=DIRECTION('ref_axis',(1.,0.,0.));
#20204=DIRECTION('center_axis',(0.,1.,0.));
#20205=DIRECTION('ref_axis',(1.,0.,0.));
#20206=DIRECTION('center_axis',(0.,-1.,0.));
#20207=DIRECTION('ref_axis',(0.987688340595138,0.,0.156434465040231));
#20208=DIRECTION('center_axis',(0.,1.,0.));
#20209=DIRECTION('ref_axis',(1.,0.,0.));
#20210=DIRECTION('center_axis',(0.,-1.,0.));
#20211=DIRECTION('ref_axis',(1.,0.,0.));
#20212=DIRECTION('center_axis',(0.,1.,0.));
#20213=DIRECTION('ref_axis',(1.,0.,0.));
#20214=DIRECTION('center_axis',(0.,-1.,0.));
#20215=DIRECTION('ref_axis',(0.987688340595138,0.,-0.156434465040231));
#20216=DIRECTION('center_axis',(0.,1.,0.));
#20217=DIRECTION('ref_axis',(1.,0.,0.));
#20218=DIRECTION('center_axis',(0.,-1.,0.));
#20219=DIRECTION('ref_axis',(0.951056516295154,0.,-0.309016994374947));
#20220=DIRECTION('center_axis',(0.,1.,0.));
#20221=DIRECTION('ref_axis',(1.,0.,0.));
#20222=DIRECTION('center_axis',(0.,-1.,0.));
#20223=DIRECTION('ref_axis',(0.891006524188368,0.,-0.453990499739547));
#20224=DIRECTION('center_axis',(0.,1.,0.));
#20225=DIRECTION('ref_axis',(1.,0.,0.));
#20226=DIRECTION('center_axis',(0.,-1.,0.));
#20227=DIRECTION('ref_axis',(0.809016994374947,0.,-0.587785252292473));
#20228=DIRECTION('center_axis',(0.,1.,0.));
#20229=DIRECTION('ref_axis',(1.,0.,0.));
#20230=DIRECTION('center_axis',(0.,-1.,0.));
#20231=DIRECTION('ref_axis',(0.707106781186548,0.,-0.707106781186547));
#20232=DIRECTION('center_axis',(0.,1.,0.));
#20233=DIRECTION('ref_axis',(1.,0.,0.));
#20234=DIRECTION('center_axis',(0.,-1.,0.));
#20235=DIRECTION('ref_axis',(0.587785252292473,0.,-0.809016994374947));
#20236=DIRECTION('center_axis',(0.,1.,0.));
#20237=DIRECTION('ref_axis',(1.,0.,0.));
#20238=DIRECTION('center_axis',(0.,-1.,0.));
#20239=DIRECTION('ref_axis',(0.453990499739547,0.,-0.891006524188368));
#20240=DIRECTION('center_axis',(0.,1.,0.));
#20241=DIRECTION('ref_axis',(1.,0.,0.));
#20242=DIRECTION('center_axis',(0.,-1.,0.));
#20243=DIRECTION('ref_axis',(0.309016994374948,0.,-0.951056516295154));
#20244=DIRECTION('center_axis',(0.,1.,0.));
#20245=DIRECTION('ref_axis',(1.,0.,0.));
#20246=DIRECTION('center_axis',(0.,-1.,0.));
#20247=DIRECTION('ref_axis',(0.156434465040231,0.,-0.987688340595138));
#20248=DIRECTION('center_axis',(0.,1.,0.));
#20249=DIRECTION('ref_axis',(1.,0.,0.));
#20250=DIRECTION('center_axis',(0.,-1.,0.));
#20251=DIRECTION('ref_axis',(6.12323399573677E-17,0.,-1.));
#20252=DIRECTION('center_axis',(0.,1.,0.));
#20253=DIRECTION('ref_axis',(1.,0.,0.));
#20254=DIRECTION('center_axis',(0.,-1.,0.));
#20255=DIRECTION('ref_axis',(-0.156434465040231,0.,-0.987688340595138));
#20256=DIRECTION('center_axis',(0.,1.,0.));
#20257=DIRECTION('ref_axis',(1.,0.,0.));
#20258=DIRECTION('center_axis',(0.,-1.,0.));
#20259=DIRECTION('ref_axis',(-0.309016994374947,0.,-0.951056516295154));
#20260=DIRECTION('center_axis',(0.,1.,0.));
#20261=DIRECTION('ref_axis',(1.,0.,0.));
#20262=DIRECTION('center_axis',(0.,-1.,0.));
#20263=DIRECTION('ref_axis',(-0.453990499739547,0.,-0.891006524188368));
#20264=DIRECTION('center_axis',(0.,1.,0.));
#20265=DIRECTION('ref_axis',(1.,0.,0.));
#20266=DIRECTION('center_axis',(0.,-1.,0.));
#20267=DIRECTION('ref_axis',(-0.587785252292473,0.,-0.809016994374947));
#20268=DIRECTION('center_axis',(0.,1.,0.));
#20269=DIRECTION('ref_axis',(1.,0.,0.));
#20270=DIRECTION('center_axis',(0.,-1.,0.));
#20271=DIRECTION('ref_axis',(-0.707106781186547,0.,-0.707106781186548));
#20272=DIRECTION('center_axis',(0.,1.,0.));
#20273=DIRECTION('ref_axis',(1.,0.,0.));
#20274=DIRECTION('center_axis',(0.,-1.,0.));
#20275=DIRECTION('ref_axis',(-0.809016994374947,0.,-0.587785252292473));
#20276=DIRECTION('center_axis',(0.,1.,0.));
#20277=DIRECTION('ref_axis',(1.,0.,0.));
#20278=DIRECTION('center_axis',(0.,-1.,0.));
#20279=DIRECTION('ref_axis',(-0.891006524188368,0.,-0.453990499739547));
#20280=DIRECTION('center_axis',(0.,1.,0.));
#20281=DIRECTION('ref_axis',(1.,0.,0.));
#20282=DIRECTION('center_axis',(0.,-1.,0.));
#20283=DIRECTION('ref_axis',(-0.951056516295154,0.,-0.309016994374948));
#20284=DIRECTION('center_axis',(0.,1.,0.));
#20285=DIRECTION('ref_axis',(1.,0.,0.));
#20286=DIRECTION('center_axis',(0.,-1.,0.));
#20287=DIRECTION('ref_axis',(-0.987688340595138,0.,-0.156434465040231));
#20288=DIRECTION('center_axis',(0.,1.,0.));
#20289=DIRECTION('ref_axis',(1.,0.,0.));
#20290=DIRECTION('center_axis',(0.,-1.,0.));
#20291=DIRECTION('ref_axis',(-1.,0.,-1.22464679914735E-16));
#20292=DIRECTION('center_axis',(0.,1.,0.));
#20293=DIRECTION('ref_axis',(1.,0.,0.));
#20294=DIRECTION('center_axis',(0.,-1.,0.));
#20295=DIRECTION('ref_axis',(-0.987688340595138,0.,0.156434465040231));
#20296=DIRECTION('center_axis',(0.,1.,0.));
#20297=DIRECTION('ref_axis',(1.,0.,0.));
#20298=DIRECTION('center_axis',(0.,-1.,0.));
#20299=DIRECTION('ref_axis',(-0.951056516295154,0.,0.309016994374947));
#20300=DIRECTION('center_axis',(0.,1.,0.));
#20301=DIRECTION('ref_axis',(1.,0.,0.));
#20302=DIRECTION('center_axis',(0.,-1.,0.));
#20303=DIRECTION('ref_axis',(-0.891006524188368,0.,0.453990499739547));
#20304=DIRECTION('center_axis',(0.,1.,0.));
#20305=DIRECTION('ref_axis',(1.,0.,0.));
#20306=DIRECTION('center_axis',(0.,-1.,0.));
#20307=DIRECTION('ref_axis',(-0.809016994374947,0.,0.587785252292473));
#20308=DIRECTION('center_axis',(0.,1.,0.));
#20309=DIRECTION('ref_axis',(1.,0.,0.));
#20310=DIRECTION('center_axis',(0.,-1.,0.));
#20311=DIRECTION('ref_axis',(-0.707106781186548,0.,0.707106781186547));
#20312=DIRECTION('center_axis',(0.,1.,0.));
#20313=DIRECTION('ref_axis',(1.,0.,0.));
#20314=DIRECTION('center_axis',(0.,-1.,0.));
#20315=DIRECTION('ref_axis',(-0.587785252292473,0.,0.809016994374947));
#20316=DIRECTION('center_axis',(0.,1.,0.));
#20317=DIRECTION('ref_axis',(1.,0.,0.));
#20318=DIRECTION('center_axis',(0.,-1.,0.));
#20319=DIRECTION('ref_axis',(-0.453990499739547,0.,0.891006524188368));
#20320=DIRECTION('center_axis',(0.,1.,0.));
#20321=DIRECTION('ref_axis',(1.,0.,0.));
#20322=DIRECTION('center_axis',(0.,-1.,0.));
#20323=DIRECTION('ref_axis',(-0.309016994374948,0.,0.951056516295154));
#20324=DIRECTION('center_axis',(0.,1.,0.));
#20325=DIRECTION('ref_axis',(1.,0.,0.));
#20326=DIRECTION('center_axis',(0.,-1.,0.));
#20327=DIRECTION('ref_axis',(-0.156434465040231,0.,0.987688340595138));
#20328=DIRECTION('center_axis',(0.,1.,0.));
#20329=DIRECTION('ref_axis',(1.,0.,0.));
#20330=DIRECTION('center_axis',(0.,-1.,0.));
#20331=DIRECTION('ref_axis',(-1.83697019872103E-16,0.,1.));
#20332=DIRECTION('center_axis',(0.,1.,0.));
#20333=DIRECTION('ref_axis',(1.,0.,0.));
#20334=DIRECTION('center_axis',(0.,-1.,0.));
#20335=DIRECTION('ref_axis',(0.156434465040231,0.,0.987688340595138));
#20336=DIRECTION('center_axis',(0.,1.,0.));
#20337=DIRECTION('ref_axis',(1.,0.,0.));
#20338=DIRECTION('center_axis',(0.,-1.,0.));
#20339=DIRECTION('ref_axis',(0.309016994374947,0.,0.951056516295154));
#20340=DIRECTION('center_axis',(0.,1.,0.));
#20341=DIRECTION('ref_axis',(1.,0.,0.));
#20342=DIRECTION('center_axis',(0.,-1.,0.));
#20343=DIRECTION('ref_axis',(0.453990499739547,0.,0.891006524188368));
#20344=DIRECTION('center_axis',(0.,1.,0.));
#20345=DIRECTION('ref_axis',(1.,0.,0.));
#20346=DIRECTION('center_axis',(0.,-1.,0.));
#20347=DIRECTION('ref_axis',(0.587785252292473,0.,0.809016994374948));
#20348=DIRECTION('center_axis',(0.,1.,0.));
#20349=DIRECTION('ref_axis',(1.,0.,0.));
#20350=DIRECTION('center_axis',(0.,-1.,0.));
#20351=DIRECTION('ref_axis',(0.707106781186547,0.,0.707106781186548));
#20352=DIRECTION('center_axis',(0.,1.,0.));
#20353=DIRECTION('ref_axis',(1.,0.,0.));
#20354=DIRECTION('center_axis',(0.,-1.,0.));
#20355=DIRECTION('ref_axis',(0.809016994374947,0.,0.587785252292473));
#20356=DIRECTION('center_axis',(0.,1.,0.));
#20357=DIRECTION('ref_axis',(1.,0.,0.));
#20358=DIRECTION('center_axis',(0.,-1.,0.));
#20359=DIRECTION('ref_axis',(0.891006524188368,0.,0.453990499739547));
#20360=DIRECTION('center_axis',(0.,1.,0.));
#20361=DIRECTION('ref_axis',(1.,0.,0.));
#20362=DIRECTION('center_axis',(0.,-1.,0.));
#20363=DIRECTION('ref_axis',(0.951056516295154,0.,0.309016994374948));
#20364=DIRECTION('center_axis',(0.,1.,0.));
#20365=DIRECTION('ref_axis',(1.,0.,0.));
#20366=DIRECTION('center_axis',(0.,1.,0.));
#20367=DIRECTION('ref_axis',(1.,0.,0.));
#20368=DIRECTION('center_axis',(0.,1.,0.));
#20369=DIRECTION('ref_axis',(1.,0.,0.));
#20370=DIRECTION('',(0.,-1.,0.));
#20371=DIRECTION('center_axis',(0.,1.,0.));
#20372=DIRECTION('ref_axis',(1.,0.,0.));
#20373=DIRECTION('center_axis',(0.,1.,0.));
#20374=DIRECTION('ref_axis',(-0.987688340595137,0.,-0.156434465040233));
#20375=DIRECTION('',(0.,-1.,0.));
#20376=DIRECTION('',(0.,1.,0.));
#20377=DIRECTION('center_axis',(0.,1.,0.));
#20378=DIRECTION('ref_axis',(1.,0.,0.));
#20379=DIRECTION('',(0.,-1.,0.));
#20380=DIRECTION('center_axis',(0.,1.,0.));
#20381=DIRECTION('ref_axis',(-0.951056516295153,0.,-0.309016994374949));
#20382=DIRECTION('',(0.,1.,0.));
#20383=DIRECTION('center_axis',(0.,1.,0.));
#20384=DIRECTION('ref_axis',(1.,0.,0.));
#20385=DIRECTION('',(0.,-1.,0.));
#20386=DIRECTION('center_axis',(0.,1.,0.));
#20387=DIRECTION('ref_axis',(-0.891006524188368,0.,-0.453990499739547));
#20388=DIRECTION('',(0.,1.,0.));
#20389=DIRECTION('center_axis',(0.,1.,0.));
#20390=DIRECTION('ref_axis',(1.,0.,0.));
#20391=DIRECTION('',(0.,-1.,0.));
#20392=DIRECTION('center_axis',(0.,1.,0.));
#20393=DIRECTION('ref_axis',(-0.809016994374948,0.,-0.587785252292473));
#20394=DIRECTION('',(0.,1.,0.));
#20395=DIRECTION('center_axis',(0.,1.,0.));
#20396=DIRECTION('ref_axis',(1.,0.,0.));
#20397=DIRECTION('',(0.,-1.,0.));
#20398=DIRECTION('center_axis',(0.,1.,0.));
#20399=DIRECTION('ref_axis',(-0.707106781186547,0.,-0.707106781186548));
#20400=DIRECTION('',(0.,1.,0.));
#20401=DIRECTION('center_axis',(0.,1.,0.));
#20402=DIRECTION('ref_axis',(1.,0.,0.));
#20403=DIRECTION('',(0.,-1.,0.));
#20404=DIRECTION('center_axis',(0.,1.,0.));
#20405=DIRECTION('ref_axis',(-0.587785252292474,0.,-0.809016994374947));
#20406=DIRECTION('',(0.,1.,0.));
#20407=DIRECTION('center_axis',(0.,1.,0.));
#20408=DIRECTION('ref_axis',(1.,0.,0.));
#20409=DIRECTION('',(0.,-1.,0.));
#20410=DIRECTION('center_axis',(0.,1.,0.));
#20411=DIRECTION('ref_axis',(-0.453990499739547,0.,-0.891006524188368));
#20412=DIRECTION('',(0.,1.,0.));
#20413=DIRECTION('center_axis',(0.,1.,0.));
#20414=DIRECTION('ref_axis',(1.,0.,0.));
#20415=DIRECTION('',(0.,-1.,0.));
#20416=DIRECTION('center_axis',(0.,1.,0.));
#20417=DIRECTION('ref_axis',(-0.309016994374948,0.,-0.951056516295153));
#20418=DIRECTION('',(0.,1.,0.));
#20419=DIRECTION('center_axis',(0.,1.,0.));
#20420=DIRECTION('ref_axis',(1.,0.,0.));
#20421=DIRECTION('',(0.,-1.,0.));
#20422=DIRECTION('center_axis',(0.,1.,0.));
#20423=DIRECTION('ref_axis',(-0.156434465040232,0.,-0.987688340595138));
#20424=DIRECTION('',(0.,1.,0.));
#20425=DIRECTION('center_axis',(0.,1.,0.));
#20426=DIRECTION('ref_axis',(1.,0.,0.));
#20427=DIRECTION('',(0.,-1.,0.));
#20428=DIRECTION('center_axis',(0.,1.,0.));
#20429=DIRECTION('ref_axis',(3.06161699786838E-16,0.,-1.));
#20430=DIRECTION('',(0.,1.,0.));
#20431=DIRECTION('center_axis',(0.,1.,0.));
#20432=DIRECTION('ref_axis',(1.,0.,0.));
#20433=DIRECTION('',(0.,-1.,0.));
#20434=DIRECTION('center_axis',(0.,1.,0.));
#20435=DIRECTION('ref_axis',(0.156434465040233,0.,-0.987688340595138));
#20436=DIRECTION('',(0.,1.,0.));
#20437=DIRECTION('center_axis',(0.,1.,0.));
#20438=DIRECTION('ref_axis',(1.,0.,0.));
#20439=DIRECTION('',(0.,-1.,0.));
#20440=DIRECTION('center_axis',(0.,1.,0.));
#20441=DIRECTION('ref_axis',(0.309016994374946,0.,-0.951056516295154));
#20442=DIRECTION('',(0.,1.,0.));
#20443=DIRECTION('center_axis',(0.,1.,0.));
#20444=DIRECTION('ref_axis',(1.,0.,0.));
#20445=DIRECTION('',(0.,-1.,0.));
#20446=DIRECTION('center_axis',(0.,1.,0.));
#20447=DIRECTION('ref_axis',(0.453990499739547,0.,-0.891006524188368));
#20448=DIRECTION('',(0.,1.,0.));
#20449=DIRECTION('center_axis',(0.,1.,0.));
#20450=DIRECTION('ref_axis',(1.,0.,0.));
#20451=DIRECTION('',(0.,-1.,0.));
#20452=DIRECTION('center_axis',(0.,1.,0.));
#20453=DIRECTION('ref_axis',(0.587785252292473,0.,-0.809016994374947));
#20454=DIRECTION('',(0.,1.,0.));
#20455=DIRECTION('center_axis',(0.,1.,0.));
#20456=DIRECTION('ref_axis',(1.,0.,0.));
#20457=DIRECTION('',(0.,-1.,0.));
#20458=DIRECTION('center_axis',(0.,1.,0.));
#20459=DIRECTION('ref_axis',(0.707106781186548,0.,-0.707106781186547));
#20460=DIRECTION('',(0.,1.,0.));
#20461=DIRECTION('center_axis',(0.,1.,0.));
#20462=DIRECTION('ref_axis',(1.,0.,0.));
#20463=DIRECTION('',(0.,-1.,0.));
#20464=DIRECTION('center_axis',(0.,1.,0.));
#20465=DIRECTION('ref_axis',(0.809016994374946,0.,-0.587785252292475));
#20466=DIRECTION('',(0.,1.,0.));
#20467=DIRECTION('center_axis',(0.,1.,0.));
#20468=DIRECTION('ref_axis',(1.,0.,0.));
#20469=DIRECTION('',(0.,-1.,0.));
#20470=DIRECTION('center_axis',(0.,1.,0.));
#20471=DIRECTION('ref_axis',(0.891006524188368,0.,-0.453990499739547));
#20472=DIRECTION('',(0.,1.,0.));
#20473=DIRECTION('center_axis',(0.,1.,0.));
#20474=DIRECTION('ref_axis',(1.,0.,0.));
#20475=DIRECTION('',(0.,-1.,0.));
#20476=DIRECTION('center_axis',(0.,1.,0.));
#20477=DIRECTION('ref_axis',(0.951056516295154,0.,-0.309016994374946));
#20478=DIRECTION('',(0.,1.,0.));
#20479=DIRECTION('center_axis',(0.,1.,0.));
#20480=DIRECTION('ref_axis',(1.,0.,0.));
#20481=DIRECTION('',(0.,-1.,0.));
#20482=DIRECTION('center_axis',(0.,1.,0.));
#20483=DIRECTION('ref_axis',(0.987688340595138,0.,-0.156434465040232));
#20484=DIRECTION('',(0.,1.,0.));
#20485=DIRECTION('center_axis',(0.,1.,0.));
#20486=DIRECTION('ref_axis',(1.,0.,0.));
#20487=DIRECTION('',(0.,-1.,0.));
#20488=DIRECTION('center_axis',(0.,1.,0.));
#20489=DIRECTION('ref_axis',(1.,0.,2.44929359829471E-16));
#20490=DIRECTION('',(0.,1.,0.));
#20491=DIRECTION('center_axis',(0.,1.,0.));
#20492=DIRECTION('ref_axis',(1.,0.,0.));
#20493=DIRECTION('',(0.,-1.,0.));
#20494=DIRECTION('center_axis',(0.,1.,0.));
#20495=DIRECTION('ref_axis',(0.987688340595137,0.,0.156434465040232));
#20496=DIRECTION('',(0.,1.,0.));
#20497=DIRECTION('center_axis',(0.,1.,0.));
#20498=DIRECTION('ref_axis',(1.,0.,0.));
#20499=DIRECTION('',(0.,-1.,0.));
#20500=DIRECTION('center_axis',(0.,1.,0.));
#20501=DIRECTION('ref_axis',(0.951056516295154,0.,0.309016994374946));
#20502=DIRECTION('',(0.,1.,0.));
#20503=DIRECTION('center_axis',(0.,1.,0.));
#20504=DIRECTION('ref_axis',(1.,0.,0.));
#20505=DIRECTION('',(0.,-1.,0.));
#20506=DIRECTION('center_axis',(0.,1.,0.));
#20507=DIRECTION('ref_axis',(0.891006524188368,0.,0.453990499739547));
#20508=DIRECTION('',(0.,1.,0.));
#20509=DIRECTION('center_axis',(0.,1.,0.));
#20510=DIRECTION('ref_axis',(1.,0.,0.));
#20511=DIRECTION('',(0.,-1.,0.));
#20512=DIRECTION('center_axis',(0.,1.,0.));
#20513=DIRECTION('ref_axis',(0.809016994374947,0.,0.587785252292473));
#20514=DIRECTION('',(0.,1.,0.));
#20515=DIRECTION('center_axis',(0.,1.,0.));
#20516=DIRECTION('ref_axis',(1.,0.,0.));
#20517=DIRECTION('',(0.,-1.,0.));
#20518=DIRECTION('center_axis',(0.,1.,0.));
#20519=DIRECTION('ref_axis',(0.707106781186547,0.,0.707106781186548));
#20520=DIRECTION('',(0.,1.,0.));
#20521=DIRECTION('center_axis',(0.,1.,0.));
#20522=DIRECTION('ref_axis',(1.,0.,0.));
#20523=DIRECTION('',(0.,-1.,0.));
#20524=DIRECTION('center_axis',(0.,1.,0.));
#20525=DIRECTION('ref_axis',(0.587785252292475,0.,0.809016994374946));
#20526=DIRECTION('',(0.,1.,0.));
#20527=DIRECTION('center_axis',(0.,1.,0.));
#20528=DIRECTION('ref_axis',(1.,0.,0.));
#20529=DIRECTION('',(0.,-1.,0.));
#20530=DIRECTION('center_axis',(0.,1.,0.));
#20531=DIRECTION('ref_axis',(0.453990499739547,0.,0.891006524188368));
#20532=DIRECTION('',(0.,1.,0.));
#20533=DIRECTION('center_axis',(0.,1.,0.));
#20534=DIRECTION('ref_axis',(1.,0.,0.));
#20535=DIRECTION('',(0.,-1.,0.));
#20536=DIRECTION('center_axis',(0.,1.,0.));
#20537=DIRECTION('ref_axis',(0.309016994374946,0.,0.951056516295154));
#20538=DIRECTION('',(0.,1.,0.));
#20539=DIRECTION('center_axis',(0.,1.,0.));
#20540=DIRECTION('ref_axis',(1.,0.,0.));
#20541=DIRECTION('',(0.,-1.,0.));
#20542=DIRECTION('center_axis',(0.,1.,0.));
#20543=DIRECTION('ref_axis',(0.156434465040232,0.,0.987688340595138));
#20544=DIRECTION('',(0.,1.,0.));
#20545=DIRECTION('center_axis',(0.,1.,0.));
#20546=DIRECTION('ref_axis',(1.,0.,0.));
#20547=DIRECTION('',(0.,-1.,0.));
#20548=DIRECTION('center_axis',(0.,1.,0.));
#20549=DIRECTION('ref_axis',(-1.83697019872103E-16,0.,1.));
#20550=DIRECTION('',(0.,1.,0.));
#20551=DIRECTION('center_axis',(0.,1.,0.));
#20552=DIRECTION('ref_axis',(1.,0.,0.));
#20553=DIRECTION('',(0.,-1.,0.));
#20554=DIRECTION('center_axis',(0.,1.,0.));
#20555=DIRECTION('ref_axis',(-0.156434465040232,0.,0.987688340595138));
#20556=DIRECTION('',(0.,1.,0.));
#20557=DIRECTION('center_axis',(0.,1.,0.));
#20558=DIRECTION('ref_axis',(1.,0.,0.));
#20559=DIRECTION('',(0.,-1.,0.));
#20560=DIRECTION('center_axis',(0.,1.,0.));
#20561=DIRECTION('ref_axis',(-0.309016994374946,0.,0.951056516295154));
#20562=DIRECTION('',(0.,1.,0.));
#20563=DIRECTION('center_axis',(0.,1.,0.));
#20564=DIRECTION('ref_axis',(1.,0.,0.));
#20565=DIRECTION('',(0.,-1.,0.));
#20566=DIRECTION('center_axis',(0.,1.,0.));
#20567=DIRECTION('ref_axis',(-0.453990499739549,0.,0.891006524188367));
#20568=DIRECTION('',(0.,1.,0.));
#20569=DIRECTION('center_axis',(0.,1.,0.));
#20570=DIRECTION('ref_axis',(1.,0.,0.));
#20571=DIRECTION('',(0.,-1.,0.));
#20572=DIRECTION('center_axis',(0.,1.,0.));
#20573=DIRECTION('ref_axis',(-0.587785252292474,0.,0.809016994374947));
#20574=DIRECTION('',(0.,1.,0.));
#20575=DIRECTION('center_axis',(0.,1.,0.));
#20576=DIRECTION('ref_axis',(1.,0.,0.));
#20577=DIRECTION('',(0.,-1.,0.));
#20578=DIRECTION('center_axis',(0.,1.,0.));
#20579=DIRECTION('ref_axis',(-0.707106781186548,0.,0.707106781186547));
#20580=DIRECTION('',(0.,1.,0.));
#20581=DIRECTION('center_axis',(0.,1.,0.));
#20582=DIRECTION('ref_axis',(1.,0.,0.));
#20583=DIRECTION('',(0.,-1.,0.));
#20584=DIRECTION('center_axis',(0.,1.,0.));
#20585=DIRECTION('ref_axis',(-0.809016994374947,0.,0.587785252292474));
#20586=DIRECTION('',(0.,1.,0.));
#20587=DIRECTION('center_axis',(0.,1.,0.));
#20588=DIRECTION('ref_axis',(1.,0.,0.));
#20589=DIRECTION('',(0.,-1.,0.));
#20590=DIRECTION('center_axis',(0.,1.,0.));
#20591=DIRECTION('ref_axis',(-0.891006524188368,0.,0.453990499739547));
#20592=DIRECTION('',(0.,1.,0.));
#20593=DIRECTION('center_axis',(0.,1.,0.));
#20594=DIRECTION('ref_axis',(1.,0.,0.));
#20595=DIRECTION('',(0.,-1.,0.));
#20596=DIRECTION('center_axis',(0.,1.,0.));
#20597=DIRECTION('ref_axis',(-0.951056516295154,0.,0.309016994374948));
#20598=DIRECTION('',(0.,1.,0.));
#20599=DIRECTION('center_axis',(0.,1.,0.));
#20600=DIRECTION('ref_axis',(1.,0.,0.));
#20601=DIRECTION('',(0.,-1.,0.));
#20602=DIRECTION('center_axis',(0.,1.,0.));
#20603=DIRECTION('ref_axis',(-0.987688340595137,0.,0.156434465040233));
#20604=DIRECTION('',(0.,1.,0.));
#20605=DIRECTION('center_axis',(0.,1.,0.));
#20606=DIRECTION('ref_axis',(1.,0.,0.));
#20607=DIRECTION('',(0.,1.,0.));
#20608=DIRECTION('center_axis',(0.,1.,0.));
#20609=DIRECTION('ref_axis',(-1.,0.,-1.22464679914735E-16));
#20610=DIRECTION('',(0.,-1.,0.));
#20611=DIRECTION('center_axis',(0.,1.,0.));
#20612=DIRECTION('ref_axis',(1.,0.,0.));
#25837=CARTESIAN_POINT('',(0.,0.,0.));
#25838=CARTESIAN_POINT('Origin',(0.,-0.5,0.));
#25839=CARTESIAN_POINT('',(-1.,-0.375,-6.12323399573677E-17));
#25840=CARTESIAN_POINT('',(-0.992156741649222,-0.5,0.125));
#25841=CARTESIAN_POINT('Ctrl Pts',(-1.,-0.375,-1.00613961606655E-16));
#25842=CARTESIAN_POINT('Ctrl Pts',(-1.,-0.375,0.0157128711428661));
#25843=CARTESIAN_POINT('Ctrl Pts',(-0.999591823858855,-0.378143583103513,
0.0324619190698278));
#25844=CARTESIAN_POINT('Ctrl Pts',(-0.998116453123232,-0.390905426591754,
0.0632545375991437));
#25845=CARTESIAN_POINT('Ctrl Pts',(-0.997070068816062,-0.400522781657727,
0.0772994769543643));
#25846=CARTESIAN_POINT('Ctrl Pts',(-0.995102104277285,-0.422700615683787,
0.0994773109804239));
#25847=CARTESIAN_POINT('Ctrl Pts',(-0.994052129228928,-0.436745514765346,
0.109094593469654));
#25848=CARTESIAN_POINT('Ctrl Pts',(-0.99256853061881,-0.467537996927464,
0.121856383722779));
#25849=CARTESIAN_POINT('Ctrl Pts',(-0.992156741649222,-0.484286997589363,
0.125));
#25850=CARTESIAN_POINT('Ctrl Pts',(-0.992156741649222,-0.5,0.125));
#25851=CARTESIAN_POINT('',(-1.,-0.625,-6.12323399573677E-17));
#25852=CARTESIAN_POINT('Ctrl Pts',(-1.,-0.625,-4.5102810375397E-17));
#25853=CARTESIAN_POINT('Ctrl Pts',(-1.,-0.625,-0.0157128711428662));
#25854=CARTESIAN_POINT('Ctrl Pts',(-0.999591823858855,-0.621856416896487,
-0.032461919069828));
#25855=CARTESIAN_POINT('Ctrl Pts',(-0.998116453123232,-0.609094573408246,
-0.0632545375991439));
#25856=CARTESIAN_POINT('Ctrl Pts',(-0.997070068816062,-0.599477218342273,
-0.0772994769543645));
#25857=CARTESIAN_POINT('Ctrl Pts',(-0.995102104277285,-0.577299384316213,
-0.0994773109804241));
#25858=CARTESIAN_POINT('Ctrl Pts',(-0.994052129228928,-0.563254485234654,
-0.109094593469655));
#25859=CARTESIAN_POINT('Ctrl Pts',(-0.99256853061881,-0.532462003072536,
-0.121856383722779));
#25860=CARTESIAN_POINT('Ctrl Pts',(-0.992156741649221,-0.515713002410637,
-0.125));
#25861=CARTESIAN_POINT('Ctrl Pts',(-0.992156741649221,-0.484286997589363,
-0.125));
#25862=CARTESIAN_POINT('Ctrl Pts',(-0.99256853061881,-0.467537996927464,
-0.121856383722779));
#25863=CARTESIAN_POINT('Ctrl Pts',(-0.994052129228928,-0.436745514765346,
-0.109094593469655));
#25864=CARTESIAN_POINT('Ctrl Pts',(-0.995102104277285,-0.422700615683787,
-0.0994773109804241));
#25865=CARTESIAN_POINT('Ctrl Pts',(-0.997070068816062,-0.400522781657728,
-0.0772994769543645));
#25866=CARTESIAN_POINT('Ctrl Pts',(-0.998116453123232,-0.390905426591754,
-0.063254537599144));
#25867=CARTESIAN_POINT('Ctrl Pts',(-0.999591823858855,-0.378143583103513,
-0.0324619190698281));
#25868=CARTESIAN_POINT('Ctrl Pts',(-1.,-0.375,-0.0157128711428663));
#25869=CARTESIAN_POINT('Ctrl Pts',(-1.,-0.375,-9.36750677027476E-17));
#25870=CARTESIAN_POINT('Ctrl Pts',(-0.992156741649222,-0.5,0.125));
#25871=CARTESIAN_POINT('Ctrl Pts',(-0.992156741649222,-0.515713002410637,
0.125));
#25872=CARTESIAN_POINT('Ctrl Pts',(-0.99256853061881,-0.532462003072536,
0.121856383722779));
#25873=CARTESIAN_POINT('Ctrl Pts',(-0.994052129228928,-0.563254485234654,
0.109094593469654));
#25874=CARTESIAN_POINT('Ctrl Pts',(-0.995102104277285,-0.577299384316213,
0.0994773109804241));
#25875=CARTESIAN_POINT('Ctrl Pts',(-0.997070068816062,-0.599477218342273,
0.0772994769543644));
#25876=CARTESIAN_POINT('Ctrl Pts',(-0.998116453123232,-0.609094573408246,
0.0632545375991438));
#25877=CARTESIAN_POINT('Ctrl Pts',(-0.999591823858855,-0.621856416896487,
0.0324619190698279));
#25878=CARTESIAN_POINT('Ctrl Pts',(-1.,-0.625,0.0157128711428661));
#25879=CARTESIAN_POINT('Ctrl Pts',(-1.,-0.625,-4.85722573273506E-17));
#25880=CARTESIAN_POINT('',(-0.586834729715275,-0.5,0.125));
#25881=CARTESIAN_POINT('',(-7.65404249467096E-18,-0.5,0.125));
#25882=CARTESIAN_POINT('',(-0.6,-0.625,1.24532753107453E-17));
#25883=CARTESIAN_POINT('Ctrl Pts',(-0.6,-0.625,-4.16333634234434E-17));
#25884=CARTESIAN_POINT('Ctrl Pts',(-0.6,-0.625,0.0157444828659572));
#25885=CARTESIAN_POINT('Ctrl Pts',(-0.599317707212167,-0.621844041497889,
0.0325072544867633));
#25886=CARTESIAN_POINT('Ctrl Pts',(-0.596852269967858,-0.609072857638709,
0.0632914182239686));
#25887=CARTESIAN_POINT('Ctrl Pts',(-0.59510289473619,-0.599460146728784,
0.077316548567853));
#25888=CARTESIAN_POINT('Ctrl Pts',(-0.591804743154611,-0.577315815675743,
0.0994608796208941));
#25889=CARTESIAN_POINT('Ctrl Pts',(-0.590038488226116,-0.563290995658393,
0.109073016834181));
#25890=CARTESIAN_POINT('Ctrl Pts',(-0.587534197873268,-0.532507913768158,
0.121843784097853));
#25891=CARTESIAN_POINT('Ctrl Pts',(-0.586834729715275,-0.515745525063995,
0.125));
#25892=CARTESIAN_POINT('Ctrl Pts',(-0.586834729715275,-0.5,0.125));
#25893=CARTESIAN_POINT('',(-0.586834729715275,-0.5,-0.125));
#25894=CARTESIAN_POINT('Ctrl Pts',(-0.586834729715275,-0.5,-0.125));
#25895=CARTESIAN_POINT('Ctrl Pts',(-0.586834729715275,-0.515745525063995,
-0.125));
#25896=CARTESIAN_POINT('Ctrl Pts',(-0.587534197873268,-0.532507913768158,
-0.121843784097853));
#25897=CARTESIAN_POINT('Ctrl Pts',(-0.590038488226116,-0.563290995658393,
-0.109073016834181));
#25898=CARTESIAN_POINT('Ctrl Pts',(-0.591804743154611,-0.577315815675743,
-0.0994608796208942));
#25899=CARTESIAN_POINT('Ctrl Pts',(-0.59510289473619,-0.599460146728784,
-0.0773165485678531));
#25900=CARTESIAN_POINT('Ctrl Pts',(-0.596852269967858,-0.609072857638709,
-0.0632914182239687));
#25901=CARTESIAN_POINT('Ctrl Pts',(-0.599317707212167,-0.621844041497889,
-0.0325072544867635));
#25902=CARTESIAN_POINT('Ctrl Pts',(-0.6,-0.625,-0.0157444828659573));
#25903=CARTESIAN_POINT('Ctrl Pts',(-0.6,-0.625,-5.20417042793042E-17));
#25904=CARTESIAN_POINT('',(-0.6,-0.375,3.50046804984438E-17));
#25905=CARTESIAN_POINT('Ctrl Pts',(-0.6,-0.375,-3.46944695195361E-18));
#25906=CARTESIAN_POINT('Ctrl Pts',(-0.6,-0.375,-0.0157444828659572));
#25907=CARTESIAN_POINT('Ctrl Pts',(-0.599317707212167,-0.378155958502111,
-0.0325072544867634));
#25908=CARTESIAN_POINT('Ctrl Pts',(-0.596852269967858,-0.390927142361291,
-0.0632914182239686));
#25909=CARTESIAN_POINT('Ctrl Pts',(-0.59510289473619,-0.400539853271216,
-0.077316548567853));
#25910=CARTESIAN_POINT('Ctrl Pts',(-0.591804743154611,-0.422684184324257,
-0.0994608796208942));
#25911=CARTESIAN_POINT('Ctrl Pts',(-0.590038488226116,-0.436709004341607,
-0.109073016834181));
#25912=CARTESIAN_POINT('Ctrl Pts',(-0.587534197873268,-0.467492086231842,
-0.121843784097853));
#25913=CARTESIAN_POINT('Ctrl Pts',(-0.586834729715275,-0.484254474936005,
-0.125));
#25914=CARTESIAN_POINT('Ctrl Pts',(-0.586834729715275,-0.5,-0.125));
#25915=CARTESIAN_POINT('Ctrl Pts',(-0.586834729715275,-0.5,0.125));
#25916=CARTESIAN_POINT('Ctrl Pts',(-0.586834729715275,-0.484254474936005,
0.125));
#25917=CARTESIAN_POINT('Ctrl Pts',(-0.587534197873268,-0.467492086231842,
0.121843784097853));
#25918=CARTESIAN_POINT('Ctrl Pts',(-0.590038488226116,-0.436709004341607,
0.109073016834181));
#25919=CARTESIAN_POINT('Ctrl Pts',(-0.591804743154611,-0.422684184324257,
0.0994608796208941));
#25920=CARTESIAN_POINT('Ctrl Pts',(-0.59510289473619,-0.400539853271216,
0.077316548567853));
#25921=CARTESIAN_POINT('Ctrl Pts',(-0.596852269967858,-0.390927142361291,
0.0632914182239686));
#25922=CARTESIAN_POINT('Ctrl Pts',(-0.599317707212167,-0.378155958502111,
0.0325072544867634));
#25923=CARTESIAN_POINT('Ctrl Pts',(-0.6,-0.375,0.0157444828659572));
#25924=CARTESIAN_POINT('Ctrl Pts',(-0.6,-0.375,-2.42861286636753E-17));
#25925=CARTESIAN_POINT('Origin',(0.,-0.5,0.));
#25926=CARTESIAN_POINT('',(0.586834729715275,-0.5,-0.125));
#25927=CARTESIAN_POINT('',(0.586834729715275,-0.5,0.125));
#25928=CARTESIAN_POINT('Ctrl Pts',(0.586834729715275,-0.5,-0.125));
#25929=CARTESIAN_POINT('Ctrl Pts',(0.586834729715275,-0.484254474936005,
-0.125));
#25930=CARTESIAN_POINT('Ctrl Pts',(0.587534197873268,-0.467492086231842,
-0.121843784097853));
#25931=CARTESIAN_POINT('Ctrl Pts',(0.590038488226116,-0.436709004341607,
-0.109073016834181));
#25932=CARTESIAN_POINT('Ctrl Pts',(0.591804743154611,-0.422684184324257,
-0.0994608796208941));
#25933=CARTESIAN_POINT('Ctrl Pts',(0.59510289473619,-0.400539853271216,
-0.0773165485678529));
#25934=CARTESIAN_POINT('Ctrl Pts',(0.596852269967858,-0.390927142361291,
-0.0632914182239686));
#25935=CARTESIAN_POINT('Ctrl Pts',(0.599317707212167,-0.378155958502111,
-0.0325072544867633));
#25936=CARTESIAN_POINT('Ctrl Pts',(0.6,-0.375,-0.0157444828659572));
#25937=CARTESIAN_POINT('Ctrl Pts',(0.6,-0.375,0.0157444828659573));
#25938=CARTESIAN_POINT('Ctrl Pts',(0.599317707212167,-0.378155958502111,
0.0325072544867635));
#25939=CARTESIAN_POINT('Ctrl Pts',(0.596852269967858,-0.390927142361291,
0.0632914182239687));
#25940=CARTESIAN_POINT('Ctrl Pts',(0.59510289473619,-0.400539853271216,
0.0773165485678531));
#25941=CARTESIAN_POINT('Ctrl Pts',(0.591804743154611,-0.422684184324257,
0.0994608796208942));
#25942=CARTESIAN_POINT('Ctrl Pts',(0.590038488226116,-0.436709004341607,
0.109073016834181));
#25943=CARTESIAN_POINT('Ctrl Pts',(0.587534197873268,-0.467492086231842,
0.121843784097853));
#25944=CARTESIAN_POINT('Ctrl Pts',(0.586834729715275,-0.484254474936005,
0.125));
#25945=CARTESIAN_POINT('Ctrl Pts',(0.586834729715275,-0.5,0.125));
#25946=CARTESIAN_POINT('Ctrl Pts',(0.586834729715275,-0.5,0.125));
#25947=CARTESIAN_POINT('Ctrl Pts',(0.586834729715275,-0.515745525063995,
0.125));
#25948=CARTESIAN_POINT('Ctrl Pts',(0.587534197873268,-0.532507913768158,
0.121843784097853));
#25949=CARTESIAN_POINT('Ctrl Pts',(0.590038488226116,-0.563290995658393,
0.109073016834181));
#25950=CARTESIAN_POINT('Ctrl Pts',(0.591804743154611,-0.577315815675743,
0.0994608796208942));
#25951=CARTESIAN_POINT('Ctrl Pts',(0.59510289473619,-0.599460146728784,
0.077316548567853));
#25952=CARTESIAN_POINT('Ctrl Pts',(0.596852269967858,-0.609072857638709,
0.0632914182239688));
#25953=CARTESIAN_POINT('Ctrl Pts',(0.599317707212167,-0.621844041497889,
0.0325072544867635));
#25954=CARTESIAN_POINT('Ctrl Pts',(0.6,-0.625,0.0157444828659573));
#25955=CARTESIAN_POINT('Ctrl Pts',(0.6,-0.625,-0.0157444828659572));
#25956=CARTESIAN_POINT('Ctrl Pts',(0.599317707212167,-0.621844041497889,
-0.0325072544867633));
#25957=CARTESIAN_POINT('Ctrl Pts',(0.596852269967858,-0.609072857638709,
-0.0632914182239685));
#25958=CARTESIAN_POINT('Ctrl Pts',(0.59510289473619,-0.599460146728784,
-0.077316548567853));
#25959=CARTESIAN_POINT('Ctrl Pts',(0.591804743154611,-0.577315815675743,
-0.0994608796208941));
#25960=CARTESIAN_POINT('Ctrl Pts',(0.590038488226116,-0.563290995658393,
-0.10907301683418));
#25961=CARTESIAN_POINT('Ctrl Pts',(0.587534197873268,-0.532507913768158,
-0.121843784097853));
#25962=CARTESIAN_POINT('Ctrl Pts',(0.586834729715275,-0.515745525063995,
-0.125));
#25963=CARTESIAN_POINT('Ctrl Pts',(0.586834729715275,-0.5,-0.125));
#25964=CARTESIAN_POINT('',(0.992156741649222,-0.5,0.125));
#25965=CARTESIAN_POINT('',(-7.65404249467096E-18,-0.5,0.125));
#25966=CARTESIAN_POINT('',(1.,-0.625,6.12323399573677E-17));
#25967=CARTESIAN_POINT('Ctrl Pts',(1.,-0.625,7.28583859910259E-17));
#25968=CARTESIAN_POINT('Ctrl Pts',(1.,-0.625,0.0157128711428663));
#25969=CARTESIAN_POINT('Ctrl Pts',(0.999591823858855,-0.621856416896487,
0.032461919069828));
#25970=CARTESIAN_POINT('Ctrl Pts',(0.998116453123232,-0.609094573408246,
0.0632545375991439));
#25971=CARTESIAN_POINT('Ctrl Pts',(0.997070068816062,-0.599477218342273,
0.0772994769543645));
#25972=CARTESIAN_POINT('Ctrl Pts',(0.995102104277285,-0.577299384316213,
0.0994773109804242));
#25973=CARTESIAN_POINT('Ctrl Pts',(0.994052129228928,-0.563254485234654,
0.109094593469655));
#25974=CARTESIAN_POINT('Ctrl Pts',(0.99256853061881,-0.532462003072536,
0.121856383722779));
#25975=CARTESIAN_POINT('Ctrl Pts',(0.992156741649222,-0.515713002410637,
0.125));
#25976=CARTESIAN_POINT('Ctrl Pts',(0.992156741649222,-0.5,0.125));
#25977=CARTESIAN_POINT('',(1.,-0.375,6.12323399573677E-17));
#25978=CARTESIAN_POINT('Ctrl Pts',(1.,-0.375,2.08166817117217E-17));
#25979=CARTESIAN_POINT('Ctrl Pts',(1.,-0.375,-0.0157128711428662));
#25980=CARTESIAN_POINT('Ctrl Pts',(0.999591823858855,-0.378143583103513,
-0.032461919069828));
#25981=CARTESIAN_POINT('Ctrl Pts',(0.998116453123232,-0.390905426591754,
-0.0632545375991438));
#25982=CARTESIAN_POINT('Ctrl Pts',(0.997070068816062,-0.400522781657728,
-0.0772994769543644));
#25983=CARTESIAN_POINT('Ctrl Pts',(0.995102104277285,-0.422700615683787,
-0.099477310980424));
#25984=CARTESIAN_POINT('Ctrl Pts',(0.994052129228928,-0.436745514765346,
-0.109094593469654));
#25985=CARTESIAN_POINT('Ctrl Pts',(0.99256853061881,-0.467537996927464,
-0.121856383722779));
#25986=CARTESIAN_POINT('Ctrl Pts',(0.992156741649222,-0.484286997589363,
-0.125));
#25987=CARTESIAN_POINT('Ctrl Pts',(0.992156741649222,-0.515713002410637,
-0.125));
#25988=CARTESIAN_POINT('Ctrl Pts',(0.99256853061881,-0.532462003072536,
-0.121856383722779));
#25989=CARTESIAN_POINT('Ctrl Pts',(0.994052129228928,-0.563254485234654,
-0.109094593469654));
#25990=CARTESIAN_POINT('Ctrl Pts',(0.995102104277285,-0.577299384316213,
-0.099477310980424));
#25991=CARTESIAN_POINT('Ctrl Pts',(0.997070068816062,-0.599477218342273,
-0.0772994769543643));
#25992=CARTESIAN_POINT('Ctrl Pts',(0.998116453123232,-0.609094573408246,
-0.0632545375991438));
#25993=CARTESIAN_POINT('Ctrl Pts',(0.999591823858855,-0.621856416896487,
-0.0324619190698279));
#25994=CARTESIAN_POINT('Ctrl Pts',(1.,-0.625,-0.0157128711428661));
#25995=CARTESIAN_POINT('Ctrl Pts',(1.,-0.625,8.32667268468867E-17));
#25996=CARTESIAN_POINT('Ctrl Pts',(0.992156741649222,-0.5,0.125));
#25997=CARTESIAN_POINT('Ctrl Pts',(0.992156741649222,-0.484286997589363,
0.125));
#25998=CARTESIAN_POINT('Ctrl Pts',(0.99256853061881,-0.467537996927464,
0.121856383722779));
#25999=CARTESIAN_POINT('Ctrl Pts',(0.994052129228928,-0.436745514765346,
0.109094593469654));
#26000=CARTESIAN_POINT('Ctrl Pts',(0.995102104277285,-0.422700615683787,
0.0994773109804241));
#26001=CARTESIAN_POINT('Ctrl Pts',(0.997070068816062,-0.400522781657727,
0.0772994769543644));
#26002=CARTESIAN_POINT('Ctrl Pts',(0.998116453123232,-0.390905426591754,
0.0632545375991438));
#26003=CARTESIAN_POINT('Ctrl Pts',(0.999591823858855,-0.378143583103513,
0.0324619190698279));
#26004=CARTESIAN_POINT('Ctrl Pts',(1.,-0.375,0.0157128711428662));
#26005=CARTESIAN_POINT('Ctrl Pts',(1.,-0.375,2.77555756156289E-17));
#26006=CARTESIAN_POINT('Origin',(0.,-0.1,0.));
#26007=CARTESIAN_POINT('',(-1.,-0.9,1.22464679914735E-16));
#26008=CARTESIAN_POINT('Origin',(0.,-0.9,0.));
#26009=CARTESIAN_POINT('',(-1.,-0.1,-1.22464679914735E-16));
#26010=CARTESIAN_POINT('',(-1.,-0.1,1.22464679914735E-16));
#26011=CARTESIAN_POINT('',(-1.,-0.1,-1.22464679914735E-16));
#26012=CARTESIAN_POINT('Origin',(0.,-0.1,0.));
#26013=CARTESIAN_POINT('',(0.,-0.625,-1.));
#26014=CARTESIAN_POINT('',(0.,-0.375,-1.));
#26015=CARTESIAN_POINT('Ctrl Pts',(-2.08166817117217E-17,-0.625,-1.));
#26016=CARTESIAN_POINT('Ctrl Pts',(0.0157128711428662,-0.625,-1.));
#26017=CARTESIAN_POINT('Ctrl Pts',(0.0324619190698279,-0.621856416896487,
-0.999591823858855));
#26018=CARTESIAN_POINT('Ctrl Pts',(0.0632545375991438,-0.609094573408246,
-0.998116453123232));
#26019=CARTESIAN_POINT('Ctrl Pts',(0.0772994769543644,-0.599477218342273,
-0.997070068816062));
#26020=CARTESIAN_POINT('Ctrl Pts',(0.0994773109804241,-0.577299384316213,
-0.995102104277285));
#26021=CARTESIAN_POINT('Ctrl Pts',(0.109094593469654,-0.563254485234654,
-0.994052129228928));
#26022=CARTESIAN_POINT('Ctrl Pts',(0.121856383722779,-0.532462003072536,
-0.99256853061881));
#26023=CARTESIAN_POINT('Ctrl Pts',(0.125,-0.515713002410637,-0.992156741649221));
#26024=CARTESIAN_POINT('Ctrl Pts',(0.125,-0.484286997589363,-0.992156741649221));
#26025=CARTESIAN_POINT('Ctrl Pts',(0.121856383722779,-0.467537996927464,
-0.99256853061881));
#26026=CARTESIAN_POINT('Ctrl Pts',(0.109094593469654,-0.436745514765346,
-0.994052129228928));
#26027=CARTESIAN_POINT('Ctrl Pts',(0.0994773109804241,-0.422700615683787,
-0.995102104277285));
#26028=CARTESIAN_POINT('Ctrl Pts',(0.0772994769543645,-0.400522781657728,
-0.997070068816062));
#26029=CARTESIAN_POINT('Ctrl Pts',(0.0632545375991439,-0.390905426591754,
-0.998116453123232));
#26030=CARTESIAN_POINT('Ctrl Pts',(0.032461919069828,-0.378143583103513,
-0.999591823858855));
#26031=CARTESIAN_POINT('Ctrl Pts',(0.0157128711428662,-0.375,-1.));
#26032=CARTESIAN_POINT('Ctrl Pts',(3.81639164714898E-17,-0.375,-1.));
#26033=CARTESIAN_POINT('',(-0.125,-0.5,-0.992156741649222));
#26034=CARTESIAN_POINT('Ctrl Pts',(4.5102810375397E-17,-0.375,-1.));
#26035=CARTESIAN_POINT('Ctrl Pts',(-0.0157128711428661,-0.375,-1.));
#26036=CARTESIAN_POINT('Ctrl Pts',(-0.0324619190698279,-0.378143583103513,
-0.999591823858855));
#26037=CARTESIAN_POINT('Ctrl Pts',(-0.0632545375991437,-0.390905426591754,
-0.998116453123232));
#26038=CARTESIAN_POINT('Ctrl Pts',(-0.0772994769543643,-0.400522781657727,
-0.997070068816062));
#26039=CARTESIAN_POINT('Ctrl Pts',(-0.099477310980424,-0.422700615683787,
-0.995102104277285));
#26040=CARTESIAN_POINT('Ctrl Pts',(-0.109094593469654,-0.436745514765346,
-0.994052129228928));
#26041=CARTESIAN_POINT('Ctrl Pts',(-0.121856383722779,-0.467537996927464,
-0.99256853061881));
#26042=CARTESIAN_POINT('Ctrl Pts',(-0.125,-0.484286997589363,-0.992156741649222));
#26043=CARTESIAN_POINT('Ctrl Pts',(-0.125,-0.5,-0.992156741649222));
#26044=CARTESIAN_POINT('Ctrl Pts',(-0.125,-0.5,-0.992156741649222));
#26045=CARTESIAN_POINT('Ctrl Pts',(-0.125,-0.515713002410637,-0.992156741649222));
#26046=CARTESIAN_POINT('Ctrl Pts',(-0.121856383722779,-0.532462003072536,
-0.99256853061881));
#26047=CARTESIAN_POINT('Ctrl Pts',(-0.109094593469654,-0.563254485234654,
-0.994052129228928));
#26048=CARTESIAN_POINT('Ctrl Pts',(-0.0994773109804241,-0.577299384316213,
-0.995102104277285));
#26049=CARTESIAN_POINT('Ctrl Pts',(-0.0772994769543644,-0.599477218342273,
-0.997070068816062));
#26050=CARTESIAN_POINT('Ctrl Pts',(-0.0632545375991439,-0.609094573408246,
-0.998116453123232));
#26051=CARTESIAN_POINT('Ctrl Pts',(-0.032461919069828,-0.621856416896487,
-0.999591823858855));
#26052=CARTESIAN_POINT('Ctrl Pts',(-0.0157128711428662,-0.625,-1.));
#26053=CARTESIAN_POINT('Ctrl Pts',(-1.38777878078145E-17,-0.625,-1.));
#26054=CARTESIAN_POINT('',(0.,-0.375,1.));
#26055=CARTESIAN_POINT('',(0.,-0.625,1.));
#26056=CARTESIAN_POINT('Ctrl Pts',(4.16333634234434E-17,-0.375,1.));
#26057=CARTESIAN_POINT('Ctrl Pts',(0.0157128711428662,-0.375,1.));
#26058=CARTESIAN_POINT('Ctrl Pts',(0.032461919069828,-0.378143583103513,
0.999591823858855));
#26059=CARTESIAN_POINT('Ctrl Pts',(0.0632545375991439,-0.390905426591754,
0.998116453123232));
#26060=CARTESIAN_POINT('Ctrl Pts',(0.0772994769543644,-0.400522781657728,
0.997070068816062));
#26061=CARTESIAN_POINT('Ctrl Pts',(0.0994773109804241,-0.422700615683787,
0.995102104277285));
#26062=CARTESIAN_POINT('Ctrl Pts',(0.109094593469654,-0.436745514765346,
0.994052129228928));
#26063=CARTESIAN_POINT('Ctrl Pts',(0.121856383722779,-0.467537996927464,
0.99256853061881));
#26064=CARTESIAN_POINT('Ctrl Pts',(0.125,-0.484286997589363,0.992156741649222));
#26065=CARTESIAN_POINT('Ctrl Pts',(0.125,-0.515713002410637,0.992156741649222));
#26066=CARTESIAN_POINT('Ctrl Pts',(0.121856383722779,-0.532462003072536,
0.99256853061881));
#26067=CARTESIAN_POINT('Ctrl Pts',(0.109094593469655,-0.563254485234654,
0.994052129228928));
#26068=CARTESIAN_POINT('Ctrl Pts',(0.0994773109804241,-0.577299384316213,
0.995102104277285));
#26069=CARTESIAN_POINT('Ctrl Pts',(0.0772994769543644,-0.599477218342273,
0.997070068816062));
#26070=CARTESIAN_POINT('Ctrl Pts',(0.0632545375991438,-0.609094573408246,
0.998116453123232));
#26071=CARTESIAN_POINT('Ctrl Pts',(0.0324619190698279,-0.621856416896487,
0.999591823858855));
#26072=CARTESIAN_POINT('Ctrl Pts',(0.0157128711428662,-0.625,1.));
#26073=CARTESIAN_POINT('Ctrl Pts',(-1.73472347597681E-17,-0.625,1.));
#26074=CARTESIAN_POINT('',(-0.125,-0.5,0.992156741649222));
#26075=CARTESIAN_POINT('Ctrl Pts',(-1.73472347597681E-17,-0.625,1.));
#26076=CARTESIAN_POINT('Ctrl Pts',(-0.0157128711428662,-0.625,1.));
#26077=CARTESIAN_POINT('Ctrl Pts',(-0.032461919069828,-0.621856416896487,
0.999591823858855));
#26078=CARTESIAN_POINT('Ctrl Pts',(-0.0632545375991439,-0.609094573408246,
0.998116453123232));
#26079=CARTESIAN_POINT('Ctrl Pts',(-0.0772994769543645,-0.599477218342273,
0.997070068816062));
#26080=CARTESIAN_POINT('Ctrl Pts',(-0.0994773109804241,-0.577299384316213,
0.995102104277285));
#26081=CARTESIAN_POINT('Ctrl Pts',(-0.109094593469654,-0.563254485234654,
0.994052129228928));
#26082=CARTESIAN_POINT('Ctrl Pts',(-0.121856383722779,-0.532462003072536,
0.99256853061881));
#26083=CARTESIAN_POINT('Ctrl Pts',(-0.125,-0.515713002410637,0.992156741649222));
#26084=CARTESIAN_POINT('Ctrl Pts',(-0.125,-0.5,0.992156741649222));
#26085=CARTESIAN_POINT('Ctrl Pts',(-0.125,-0.5,0.992156741649222));
#26086=CARTESIAN_POINT('Ctrl Pts',(-0.125,-0.484286997589363,0.992156741649222));
#26087=CARTESIAN_POINT('Ctrl Pts',(-0.121856383722779,-0.467537996927464,
0.99256853061881));
#26088=CARTESIAN_POINT('Ctrl Pts',(-0.109094593469654,-0.436745514765346,
0.994052129228928));
#26089=CARTESIAN_POINT('Ctrl Pts',(-0.099477310980424,-0.422700615683787,
0.995102104277285));
#26090=CARTESIAN_POINT('Ctrl Pts',(-0.0772994769543643,-0.400522781657727,
0.997070068816062));
#26091=CARTESIAN_POINT('Ctrl Pts',(-0.0632545375991438,-0.390905426591754,
0.998116453123232));
#26092=CARTESIAN_POINT('Ctrl Pts',(-0.0324619190698279,-0.378143583103513,
0.999591823858855));
#26093=CARTESIAN_POINT('Ctrl Pts',(-0.0157128711428661,-0.375,1.));
#26094=CARTESIAN_POINT('Ctrl Pts',(4.5102810375397E-17,-0.375,1.));
#26095=CARTESIAN_POINT('Origin',(0.,-0.5,0.));
#26096=CARTESIAN_POINT('',(-0.125,-0.5,-0.586834729715275));
#26097=CARTESIAN_POINT('',(-0.125,-0.5,0.));
#26098=CARTESIAN_POINT('',(0.125,-0.5,-0.586834729715275));
#26099=CARTESIAN_POINT('Ctrl Pts',(0.125,-0.5,-0.586834729715275));
#26100=CARTESIAN_POINT('Ctrl Pts',(0.125,-0.515745525063995,-0.586834729715275));
#26101=CARTESIAN_POINT('Ctrl Pts',(0.121843784097853,-0.532507913768158,
-0.587534197873268));
#26102=CARTESIAN_POINT('Ctrl Pts',(0.109073016834181,-0.563290995658393,
-0.590038488226116));
#26103=CARTESIAN_POINT('Ctrl Pts',(0.0994608796208942,-0.577315815675743,
-0.591804743154611));
#26104=CARTESIAN_POINT('Ctrl Pts',(0.077316548567853,-0.599460146728784,
-0.59510289473619));
#26105=CARTESIAN_POINT('Ctrl Pts',(0.0632914182239686,-0.609072857638709,
-0.596852269967858));
#26106=CARTESIAN_POINT('Ctrl Pts',(0.0325072544867633,-0.621844041497889,
-0.599317707212167));
#26107=CARTESIAN_POINT('Ctrl Pts',(0.0157444828659573,-0.625,-0.6));
#26108=CARTESIAN_POINT('Ctrl Pts',(-0.0157444828659572,-0.625,-0.6));
#26109=CARTESIAN_POINT('Ctrl Pts',(-0.0325072544867633,-0.621844041497889,
-0.599317707212167));
#26110=CARTESIAN_POINT('Ctrl Pts',(-0.0632914182239686,-0.609072857638709,
-0.596852269967858));
#26111=CARTESIAN_POINT('Ctrl Pts',(-0.077316548567853,-0.599460146728784,
-0.59510289473619));
#26112=CARTESIAN_POINT('Ctrl Pts',(-0.0994608796208941,-0.577315815675743,
-0.591804743154611));
#26113=CARTESIAN_POINT('Ctrl Pts',(-0.109073016834181,-0.563290995658393,
-0.590038488226116));
#26114=CARTESIAN_POINT('Ctrl Pts',(-0.121843784097853,-0.532507913768158,
-0.587534197873268));
#26115=CARTESIAN_POINT('Ctrl Pts',(-0.125,-0.515745525063995,-0.586834729715275));
#26116=CARTESIAN_POINT('Ctrl Pts',(-0.125,-0.5,-0.586834729715275));
#26117=CARTESIAN_POINT('Ctrl Pts',(-0.125,-0.5,-0.586834729715275));
#26118=CARTESIAN_POINT('Ctrl Pts',(-0.125,-0.484254474936005,-0.586834729715275));
#26119=CARTESIAN_POINT('Ctrl Pts',(-0.121843784097853,-0.467492086231842,
-0.587534197873268));
#26120=CARTESIAN_POINT('Ctrl Pts',(-0.109073016834181,-0.436709004341607,
-0.590038488226116));
#26121=CARTESIAN_POINT('Ctrl Pts',(-0.0994608796208942,-0.422684184324257,
-0.591804743154611));
#26122=CARTESIAN_POINT('Ctrl Pts',(-0.077316548567853,-0.400539853271216,
-0.59510289473619));
#26123=CARTESIAN_POINT('Ctrl Pts',(-0.0632914182239687,-0.39092714236129,
-0.596852269967858));
#26124=CARTESIAN_POINT('Ctrl Pts',(-0.0325072544867634,-0.378155958502111,
-0.599317707212167));
#26125=CARTESIAN_POINT('Ctrl Pts',(-0.0157444828659573,-0.375,-0.6));
#26126=CARTESIAN_POINT('Ctrl Pts',(0.0157444828659572,-0.375,-0.6));
#26127=CARTESIAN_POINT('Ctrl Pts',(0.0325072544867634,-0.378155958502111,
-0.599317707212167));
#26128=CARTESIAN_POINT('Ctrl Pts',(0.0632914182239686,-0.390927142361291,
-0.596852269967858));
#26129=CARTESIAN_POINT('Ctrl Pts',(0.077316548567853,-0.400539853271216,
-0.59510289473619));
#26130=CARTESIAN_POINT('Ctrl Pts',(0.0994608796208941,-0.422684184324257,
-0.591804743154611));
#26131=CARTESIAN_POINT('Ctrl Pts',(0.109073016834181,-0.436709004341607,
-0.590038488226116));
#26132=CARTESIAN_POINT('Ctrl Pts',(0.121843784097853,-0.467492086231842,
-0.587534197873268));
#26133=CARTESIAN_POINT('Ctrl Pts',(0.125,-0.484254474936005,-0.586834729715275));
#26134=CARTESIAN_POINT('Ctrl Pts',(0.125,-0.5,-0.586834729715275));
#26135=CARTESIAN_POINT('Origin',(0.,-0.5,0.));
#26136=CARTESIAN_POINT('',(0.125,-0.5,0.586834729715275));
#26137=CARTESIAN_POINT('',(-0.125,-0.5,0.586834729715275));
#26138=CARTESIAN_POINT('Ctrl Pts',(0.125,-0.5,0.586834729715275));
#26139=CARTESIAN_POINT('Ctrl Pts',(0.125,-0.484254474936005,0.586834729715275));
#26140=CARTESIAN_POINT('Ctrl Pts',(0.121843784097853,-0.467492086231842,
0.587534197873268));
#26141=CARTESIAN_POINT('Ctrl Pts',(0.109073016834181,-0.436709004341607,
0.590038488226116));
#26142=CARTESIAN_POINT('Ctrl Pts',(0.0994608796208941,-0.422684184324257,
0.591804743154611));
#26143=CARTESIAN_POINT('Ctrl Pts',(0.077316548567853,-0.400539853271216,
0.59510289473619));
#26144=CARTESIAN_POINT('Ctrl Pts',(0.0632914182239686,-0.390927142361291,
0.596852269967858));
#26145=CARTESIAN_POINT('Ctrl Pts',(0.0325072544867634,-0.378155958502111,
0.599317707212167));
#26146=CARTESIAN_POINT('Ctrl Pts',(0.0157444828659572,-0.375,0.6));
#26147=CARTESIAN_POINT('Ctrl Pts',(-0.0157444828659573,-0.375,0.6));
#26148=CARTESIAN_POINT('Ctrl Pts',(-0.0325072544867634,-0.378155958502111,
0.599317707212167));
#26149=CARTESIAN_POINT('Ctrl Pts',(-0.0632914182239687,-0.390927142361291,
0.596852269967858));
#26150=CARTESIAN_POINT('Ctrl Pts',(-0.077316548567853,-0.400539853271216,
0.59510289473619));
#26151=CARTESIAN_POINT('Ctrl Pts',(-0.0994608796208942,-0.422684184324257,
0.591804743154611));
#26152=CARTESIAN_POINT('Ctrl Pts',(-0.109073016834181,-0.436709004341607,
0.590038488226116));
#26153=CARTESIAN_POINT('Ctrl Pts',(-0.121843784097853,-0.467492086231842,
0.587534197873268));
#26154=CARTESIAN_POINT('Ctrl Pts',(-0.125,-0.484254474936005,0.586834729715275));
#26155=CARTESIAN_POINT('Ctrl Pts',(-0.125,-0.5,0.586834729715275));
#26156=CARTESIAN_POINT('Ctrl Pts',(-0.125,-0.5,0.586834729715275));
#26157=CARTESIAN_POINT('Ctrl Pts',(-0.125,-0.515745525063995,0.586834729715275));
#26158=CARTESIAN_POINT('Ctrl Pts',(-0.121843784097853,-0.532507913768158,
0.587534197873268));
#26159=CARTESIAN_POINT('Ctrl Pts',(-0.109073016834181,-0.563290995658393,
0.590038488226116));
#26160=CARTESIAN_POINT('Ctrl Pts',(-0.0994608796208941,-0.577315815675743,
0.591804743154611));
#26161=CARTESIAN_POINT('Ctrl Pts',(-0.077316548567853,-0.599460146728784,
0.59510289473619));
#26162=CARTESIAN_POINT('Ctrl Pts',(-0.0632914182239687,-0.609072857638709,
0.596852269967858));
#26163=CARTESIAN_POINT('Ctrl Pts',(-0.0325072544867635,-0.621844041497889,
0.599317707212167));
#26164=CARTESIAN_POINT('Ctrl Pts',(-0.0157444828659572,-0.625,0.6));
#26165=CARTESIAN_POINT('Ctrl Pts',(0.0157444828659572,-0.625,0.6));
#26166=CARTESIAN_POINT('Ctrl Pts',(0.0325072544867633,-0.621844041497889,
0.599317707212167));
#26167=CARTESIAN_POINT('Ctrl Pts',(0.0632914182239686,-0.609072857638709,
0.596852269967858));
#26168=CARTESIAN_POINT('Ctrl Pts',(0.077316548567853,-0.599460146728784,
0.59510289473619));
#26169=CARTESIAN_POINT('Ctrl Pts',(0.0994608796208942,-0.577315815675743,
0.591804743154611));
#26170=CARTESIAN_POINT('Ctrl Pts',(0.109073016834181,-0.563290995658393,
0.590038488226116));
#26171=CARTESIAN_POINT('Ctrl Pts',(0.121843784097853,-0.532507913768158,
0.587534197873268));
#26172=CARTESIAN_POINT('Ctrl Pts',(0.125,-0.515745525063995,0.586834729715275));
#26173=CARTESIAN_POINT('Ctrl Pts',(0.125,-0.5,0.586834729715275));
#26174=CARTESIAN_POINT('',(-0.125,-0.5,0.));
#26175=CARTESIAN_POINT('Origin',(0.,0.,0.));
#26176=CARTESIAN_POINT('',(-0.6,-0.9,7.34788079488412E-17));
#26177=CARTESIAN_POINT('Origin',(0.,-0.9,0.));
#26178=CARTESIAN_POINT('',(-0.6,0.,7.34788079488412E-17));
#26179=CARTESIAN_POINT('',(-0.6,0.85,-7.34788079488412E-17));
#26180=CARTESIAN_POINT('',(-0.6,0.,7.34788079488412E-17));
#26181=CARTESIAN_POINT('Origin',(0.,0.85,0.));
#26182=CARTESIAN_POINT('Origin',(0.,-0.9,0.));
#26183=CARTESIAN_POINT('Origin',(0.,0.,0.));
#26184=CARTESIAN_POINT('',(-1.4,0.,1.71450551880629E-16));
#26185=CARTESIAN_POINT('Origin',(0.,0.,0.));
#26186=CARTESIAN_POINT('',(1.23958209161204,0.,0.143317017690053));
#26187=CARTESIAN_POINT('',(1.22320001975977,0.,0.246749348660852));
#26188=CARTESIAN_POINT('Origin',(1.21321664662686,0.,0.192154639568406));
#26189=CARTESIAN_POINT('',(1.20190105810224,0.,0.335465908756113));
#26190=CARTESIAN_POINT('Origin',(0.,0.,0.));
#26191=CARTESIAN_POINT('',(1.16954029537568,0.,0.435062095450087));
#26192=CARTESIAN_POINT('Origin',(1.1682203282434,0.,0.379577794185952));
#26193=CARTESIAN_POINT('',(1.13462523166105,0.,0.519354515801077));
#26194=CARTESIAN_POINT('Origin',(0.,0.,0.));
#26195=CARTESIAN_POINT('',(1.08708260743774,0.,0.612662169561029));
#26196=CARTESIAN_POINT('Origin',(1.0944585482776,0.,0.557654483764164));
#26197=CARTESIAN_POINT('',(1.0394111664111,0.,0.690454891028201));
#26198=CARTESIAN_POINT('Origin',(0.,0.,0.));
#26199=CARTESIAN_POINT('',(0.977857337884349,0.,0.775176467748211));
#26200=CARTESIAN_POINT('Origin',(0.993747566553533,0.,0.72199986920298));
#26201=CARTESIAN_POINT('',(0.918603348636233,0.,0.844553975349804));
#26202=CARTESIAN_POINT('Origin',(0.,0.,0.));
#26203=CARTESIAN_POINT('',(0.844553975349804,0.,0.918603348636233));
#26204=CARTESIAN_POINT('Origin',(0.86856722168183,0.,0.86856722168183));
#26205=CARTESIAN_POINT('',(0.775176467748211,0.,0.977857337884349));
#26206=CARTESIAN_POINT('Origin',(0.,0.,0.));
#26207=CARTESIAN_POINT('',(0.690454891028201,0.,1.0394111664111));
#26208=CARTESIAN_POINT('Origin',(0.721999869202979,0.,0.993747566553533));
#26209=CARTESIAN_POINT('',(0.612662169561028,0.,1.08708260743774));
#26210=CARTESIAN_POINT('Origin',(0.,0.,0.));
#26211=CARTESIAN_POINT('',(0.519354515801077,0.,1.13462523166105));
#26212=CARTESIAN_POINT('Origin',(0.557654483764164,0.,1.0944585482776));
#26213=CARTESIAN_POINT('',(0.435062095450087,0.,1.16954029537568));
#26214=CARTESIAN_POINT('Origin',(0.,0.,0.));
#26215=CARTESIAN_POINT('',(0.335465908756113,0.,1.20190105810224));
#26216=CARTESIAN_POINT('Origin',(0.379577794185951,0.,1.1682203282434));
#26217=CARTESIAN_POINT('',(0.246749348660851,0.,1.22320001975977));
#26218=CARTESIAN_POINT('Origin',(0.,0.,0.));
#26219=CARTESIAN_POINT('',(0.143317017690053,0.,1.23958209161204));
#26220=CARTESIAN_POINT('Origin',(0.192154639568406,0.,1.21321664662686));
#26221=CARTESIAN_POINT('',(0.0523608139934478,0.,1.24674050008925));
#26222=CARTESIAN_POINT('Origin',(0.,0.,0.));
#26223=CARTESIAN_POINT('',(-0.0523608139934483,0.,1.24674050008925));
#26224=CARTESIAN_POINT('Origin',(-2.25642313758905E-16,0.,1.22833954473516));
#26225=CARTESIAN_POINT('',(-0.143317017690053,0.,1.23958209161204));
#26226=CARTESIAN_POINT('Origin',(0.,0.,0.));
#26227=CARTESIAN_POINT('',(-0.246749348660852,0.,1.22320001975977));
#26228=CARTESIAN_POINT('Origin',(-0.192154639568406,0.,1.21321664662686));
#26229=CARTESIAN_POINT('',(-0.335465908756113,0.,1.20190105810224));
#26230=CARTESIAN_POINT('Origin',(0.,0.,0.));
#26231=CARTESIAN_POINT('',(-0.435062095450087,0.,1.16954029537568));
#26232=CARTESIAN_POINT('Origin',(-0.379577794185951,0.,1.1682203282434));
#26233=CARTESIAN_POINT('',(-0.519354515801077,0.,1.13462523166105));
#26234=CARTESIAN_POINT('Origin',(0.,0.,0.));
#26235=CARTESIAN_POINT('',(-0.612662169561029,0.,1.08708260743774));
#26236=CARTESIAN_POINT('Origin',(-0.557654483764164,0.,1.0944585482776));
#26237=CARTESIAN_POINT('',(-0.690454891028201,0.,1.0394111664111));
#26238=CARTESIAN_POINT('Origin',(0.,0.,0.));
#26239=CARTESIAN_POINT('',(-0.775176467748211,0.,0.977857337884349));
#26240=CARTESIAN_POINT('Origin',(-0.721999869202979,0.,0.993747566553533));
#26241=CARTESIAN_POINT('',(-0.844553975349804,0.,0.918603348636233));
#26242=CARTESIAN_POINT('Origin',(0.,0.,0.));
#26243=CARTESIAN_POINT('',(-0.918603348636233,0.,0.844553975349804));
#26244=CARTESIAN_POINT('Origin',(-0.86856722168183,0.,0.86856722168183));
#26245=CARTESIAN_POINT('',(-0.977857337884348,0.,0.775176467748211));
#26246=CARTESIAN_POINT('Origin',(0.,0.,0.));
#26247=CARTESIAN_POINT('',(-1.0394111664111,0.,0.690454891028201));
#26248=CARTESIAN_POINT('Origin',(-0.993747566553533,0.,0.721999869202979));
#26249=CARTESIAN_POINT('',(-1.08708260743774,0.,0.612662169561028));
#26250=CARTESIAN_POINT('Origin',(0.,0.,0.));
#26251=CARTESIAN_POINT('',(-1.13462523166105,0.,0.519354515801077));
#26252=CARTESIAN_POINT('Origin',(-1.0944585482776,0.,0.557654483764164));
#26253=CARTESIAN_POINT('',(-1.16954029537568,0.,0.435062095450087));
#26254=CARTESIAN_POINT('Origin',(0.,0.,0.));
#26255=CARTESIAN_POINT('',(-1.20190105810224,0.,0.335465908756113));
#26256=CARTESIAN_POINT('Origin',(-1.1682203282434,0.,0.379577794185951));
#26257=CARTESIAN_POINT('',(-1.22320001975977,0.,0.246749348660851));
#26258=CARTESIAN_POINT('Origin',(0.,0.,0.));
#26259=CARTESIAN_POINT('',(-1.23958209161204,0.,0.143317017690053));
#26260=CARTESIAN_POINT('Origin',(-1.21321664662686,0.,0.192154639568406));
#26261=CARTESIAN_POINT('',(-1.24674050008925,0.,0.0523608139934479));
#26262=CARTESIAN_POINT('Origin',(0.,0.,0.));
#26263=CARTESIAN_POINT('',(-1.24674050008925,0.,-0.0523608139934482));
#26264=CARTESIAN_POINT('Origin',(-1.22833954473516,0.,-1.50428209172603E-16));
#26265=CARTESIAN_POINT('',(-1.23958209161204,0.,-0.143317017690053));
#26266=CARTESIAN_POINT('Origin',(0.,0.,0.));
#26267=CARTESIAN_POINT('',(-1.22320001975977,0.,-0.246749348660852));
#26268=CARTESIAN_POINT('Origin',(-1.21321664662686,0.,-0.192154639568406));
#26269=CARTESIAN_POINT('',(-1.20190105810224,0.,-0.335465908756113));
#26270=CARTESIAN_POINT('Origin',(0.,0.,0.));
#26271=CARTESIAN_POINT('',(-1.16954029537568,0.,-0.435062095450087));
#26272=CARTESIAN_POINT('Origin',(-1.1682203282434,0.,-0.379577794185951));
#26273=CARTESIAN_POINT('',(-1.13462523166105,0.,-0.519354515801077));
#26274=CARTESIAN_POINT('Origin',(0.,0.,0.));
#26275=CARTESIAN_POINT('',(-1.08708260743774,0.,-0.612662169561029));
#26276=CARTESIAN_POINT('Origin',(-1.0944585482776,0.,-0.557654483764164));
#26277=CARTESIAN_POINT('',(-1.0394111664111,0.,-0.690454891028201));
#26278=CARTESIAN_POINT('Origin',(0.,0.,0.));
#26279=CARTESIAN_POINT('',(-0.977857337884349,0.,-0.775176467748211));
#26280=CARTESIAN_POINT('Origin',(-0.993747566553533,0.,-0.721999869202979));
#26281=CARTESIAN_POINT('',(-0.918603348636233,0.,-0.844553975349804));
#26282=CARTESIAN_POINT('Origin',(0.,0.,0.));
#26283=CARTESIAN_POINT('',(-0.844553975349804,0.,-0.918603348636233));
#26284=CARTESIAN_POINT('Origin',(-0.86856722168183,0.,-0.86856722168183));
#26285=CARTESIAN_POINT('',(-0.775176467748211,0.,-0.977857337884348));
#26286=CARTESIAN_POINT('Origin',(0.,0.,0.));
#26287=CARTESIAN_POINT('',(-0.690454891028201,0.,-1.0394111664111));
#26288=CARTESIAN_POINT('Origin',(-0.721999869202979,0.,-0.993747566553533));
#26289=CARTESIAN_POINT('',(-0.612662169561028,0.,-1.08708260743774));
#26290=CARTESIAN_POINT('Origin',(0.,0.,0.));
#26291=CARTESIAN_POINT('',(-0.519354515801077,0.,-1.13462523166105));
#26292=CARTESIAN_POINT('Origin',(-0.557654483764164,0.,-1.0944585482776));
#26293=CARTESIAN_POINT('',(-0.435062095450087,0.,-1.16954029537568));
#26294=CARTESIAN_POINT('Origin',(0.,0.,0.));
#26295=CARTESIAN_POINT('',(-0.335465908756113,0.,-1.20190105810224));
#26296=CARTESIAN_POINT('Origin',(-0.379577794185951,0.,-1.1682203282434));
#26297=CARTESIAN_POINT('',(-0.246749348660852,0.,-1.22320001975977));
#26298=CARTESIAN_POINT('Origin',(0.,0.,0.));
#26299=CARTESIAN_POINT('',(-0.143317017690053,0.,-1.23958209161204));
#26300=CARTESIAN_POINT('Origin',(-0.192154639568406,0.,-1.21321664662686));
#26301=CARTESIAN_POINT('',(-0.0523608139934479,0.,-1.24674050008925));
#26302=CARTESIAN_POINT('Origin',(0.,0.,0.));
#26303=CARTESIAN_POINT('',(0.0523608139934481,0.,-1.24674050008925));
#26304=CARTESIAN_POINT('Origin',(7.52141045863017E-17,0.,-1.22833954473516));
#26305=CARTESIAN_POINT('',(0.143317017690053,0.,-1.23958209161204));
#26306=CARTESIAN_POINT('Origin',(0.,0.,0.));
#26307=CARTESIAN_POINT('',(0.246749348660852,0.,-1.22320001975977));
#26308=CARTESIAN_POINT('Origin',(0.192154639568406,0.,-1.21321664662686));
#26309=CARTESIAN_POINT('',(0.335465908756113,0.,-1.20190105810224));
#26310=CARTESIAN_POINT('Origin',(0.,0.,0.));
#26311=CARTESIAN_POINT('',(0.435062095450087,0.,-1.16954029537568));
#26312=CARTESIAN_POINT('Origin',(0.379577794185951,0.,-1.1682203282434));
#26313=CARTESIAN_POINT('',(0.519354515801077,0.,-1.13462523166105));
#26314=CARTESIAN_POINT('Origin',(0.,0.,0.));
#26315=CARTESIAN_POINT('',(0.612662169561028,0.,-1.08708260743774));
#26316=CARTESIAN_POINT('Origin',(0.557654483764164,0.,-1.0944585482776));
#26317=CARTESIAN_POINT('',(0.690454891028201,0.,-1.0394111664111));
#26318=CARTESIAN_POINT('Origin',(0.,0.,0.));
#26319=CARTESIAN_POINT('',(0.775176467748211,0.,-0.977857337884349));
#26320=CARTESIAN_POINT('Origin',(0.721999869202979,0.,-0.993747566553533));
#26321=CARTESIAN_POINT('',(0.844553975349804,0.,-0.918603348636233));
#26322=CARTESIAN_POINT('Origin',(0.,0.,0.));
#26323=CARTESIAN_POINT('',(0.918603348636233,0.,-0.844553975349804));
#26324=CARTESIAN_POINT('Origin',(0.86856722168183,0.,-0.86856722168183));
#26325=CARTESIAN_POINT('',(0.977857337884349,0.,-0.775176467748211));
#26326=CARTESIAN_POINT('Origin',(0.,0.,0.));
#26327=CARTESIAN_POINT('',(1.0394111664111,0.,-0.690454891028201));
#26328=CARTESIAN_POINT('Origin',(0.993747566553533,0.,-0.721999869202979));
#26329=CARTESIAN_POINT('',(1.08708260743774,0.,-0.612662169561028));
#26330=CARTESIAN_POINT('Origin',(0.,0.,0.));
#26331=CARTESIAN_POINT('',(1.13462523166105,0.,-0.519354515801077));
#26332=CARTESIAN_POINT('Origin',(1.0944585482776,0.,-0.557654483764164));
#26333=CARTESIAN_POINT('',(1.16954029537568,0.,-0.43506209545009));
#26334=CARTESIAN_POINT('Origin',(0.,0.,0.));
#26335=CARTESIAN_POINT('',(1.20190105810224,0.,-0.33546590875611));
#26336=CARTESIAN_POINT('Origin',(1.1682203282434,0.,-0.379577794185951));
#26337=CARTESIAN_POINT('',(1.22320001975977,0.,-0.246749348660852));
#26338=CARTESIAN_POINT('Origin',(0.,0.,0.));
#26339=CARTESIAN_POINT('',(1.23958209161204,0.,-0.143317017690053));
#26340=CARTESIAN_POINT('Origin',(1.21321664662686,0.,-0.192154639568406));
#26341=CARTESIAN_POINT('',(1.24674050008925,0.,-0.052360813993451));
#26342=CARTESIAN_POINT('Origin',(0.,0.,0.));
#26343=CARTESIAN_POINT('',(1.24674050008925,0.,0.052360813993451));
#26344=CARTESIAN_POINT('Origin',(1.22833954473516,0.,0.));
#26345=CARTESIAN_POINT('Origin',(0.,0.,0.));
#26346=CARTESIAN_POINT('Origin',(0.,0.,0.));
#26347=CARTESIAN_POINT('',(-1.4,-0.1,1.71450551880629E-16));
#26348=CARTESIAN_POINT('Origin',(0.,-0.1,0.));
#26349=CARTESIAN_POINT('',(-1.4,0.,-1.71450551880629E-16));
#26350=CARTESIAN_POINT('Origin',(0.,-0.1,0.));
#26351=CARTESIAN_POINT('Origin',(0.,0.75,0.));
#26352=CARTESIAN_POINT('',(-1.4,0.75,1.71450551880629E-16));
#26353=CARTESIAN_POINT('Origin',(0.,0.75,0.));
#26354=CARTESIAN_POINT('',(1.22320001975977,0.75,0.246749348660852));
#26355=CARTESIAN_POINT('',(1.23958209161204,0.75,0.143317017690053));
#26356=CARTESIAN_POINT('Origin',(1.21321664662686,0.75,0.192154639568406));
#26357=CARTESIAN_POINT('',(1.24674050008925,0.75,0.052360813993448));
#26358=CARTESIAN_POINT('Origin',(0.,0.75,0.));
#26359=CARTESIAN_POINT('',(1.24674050008925,0.75,-0.052360813993448));
#26360=CARTESIAN_POINT('Origin',(1.22833954473516,0.75,0.));
#26361=CARTESIAN_POINT('',(1.23958209161204,0.75,-0.143317017690053));
#26362=CARTESIAN_POINT('Origin',(0.,0.75,0.));
#26363=CARTESIAN_POINT('',(1.22320001975977,0.75,-0.246749348660852));
#26364=CARTESIAN_POINT('Origin',(1.21321664662686,0.75,-0.192154639568406));
#26365=CARTESIAN_POINT('',(1.20190105810224,0.75,-0.335465908756113));
#26366=CARTESIAN_POINT('Origin',(0.,0.75,0.));
#26367=CARTESIAN_POINT('',(1.16954029537568,0.75,-0.435062095450087));
#26368=CARTESIAN_POINT('Origin',(1.1682203282434,0.75,-0.379577794185951));
#26369=CARTESIAN_POINT('',(1.13462523166105,0.75,-0.519354515801077));
#26370=CARTESIAN_POINT('Origin',(0.,0.75,0.));
#26371=CARTESIAN_POINT('',(1.08708260743774,0.75,-0.612662169561028));
#26372=CARTESIAN_POINT('Origin',(1.0944585482776,0.75,-0.557654483764164));
#26373=CARTESIAN_POINT('',(1.0394111664111,0.75,-0.690454891028201));
#26374=CARTESIAN_POINT('Origin',(0.,0.75,0.));
#26375=CARTESIAN_POINT('',(0.977857337884349,0.75,-0.775176467748211));
#26376=CARTESIAN_POINT('Origin',(0.993747566553533,0.75,-0.721999869202979));
#26377=CARTESIAN_POINT('',(0.918603348636233,0.75,-0.844553975349804));
#26378=CARTESIAN_POINT('Origin',(0.,0.75,0.));
#26379=CARTESIAN_POINT('',(0.844553975349804,0.75,-0.918603348636233));
#26380=CARTESIAN_POINT('Origin',(0.86856722168183,0.75,-0.86856722168183));
#26381=CARTESIAN_POINT('',(0.775176467748211,0.75,-0.977857337884349));
#26382=CARTESIAN_POINT('Origin',(0.,0.75,0.));
#26383=CARTESIAN_POINT('',(0.690454891028201,0.75,-1.0394111664111));
#26384=CARTESIAN_POINT('Origin',(0.721999869202979,0.75,-0.993747566553533));
#26385=CARTESIAN_POINT('',(0.612662169561028,0.75,-1.08708260743774));
#26386=CARTESIAN_POINT('Origin',(0.,0.75,0.));
#26387=CARTESIAN_POINT('',(0.519354515801077,0.75,-1.13462523166105));
#26388=CARTESIAN_POINT('Origin',(0.557654483764164,0.75,-1.0944585482776));
#26389=CARTESIAN_POINT('',(0.435062095450087,0.75,-1.16954029537568));
#26390=CARTESIAN_POINT('Origin',(0.,0.75,0.));
#26391=CARTESIAN_POINT('',(0.335465908756113,0.75,-1.20190105810224));
#26392=CARTESIAN_POINT('Origin',(0.379577794185951,0.75,-1.1682203282434));
#26393=CARTESIAN_POINT('',(0.246749348660852,0.75,-1.22320001975977));
#26394=CARTESIAN_POINT('Origin',(0.,0.75,0.));
#26395=CARTESIAN_POINT('',(0.143317017690053,0.75,-1.23958209161204));
#26396=CARTESIAN_POINT('Origin',(0.192154639568406,0.75,-1.21321664662686));
#26397=CARTESIAN_POINT('',(0.0523608139934481,0.75,-1.24674050008925));
#26398=CARTESIAN_POINT('Origin',(0.,0.75,0.));
#26399=CARTESIAN_POINT('',(-0.0523608139934479,0.75,-1.24674050008925));
#26400=CARTESIAN_POINT('Origin',(7.52141045863017E-17,0.75,-1.22833954473516));
#26401=CARTESIAN_POINT('',(-0.143317017690053,0.75,-1.23958209161204));
#26402=CARTESIAN_POINT('Origin',(0.,0.75,0.));
#26403=CARTESIAN_POINT('',(-0.246749348660852,0.75,-1.22320001975977));
#26404=CARTESIAN_POINT('Origin',(-0.192154639568406,0.75,-1.21321664662686));
#26405=CARTESIAN_POINT('',(-0.335465908756113,0.75,-1.20190105810224));
#26406=CARTESIAN_POINT('Origin',(0.,0.75,0.));
#26407=CARTESIAN_POINT('',(-0.435062095450087,0.75,-1.16954029537568));
#26408=CARTESIAN_POINT('Origin',(-0.379577794185951,0.75,-1.1682203282434));
#26409=CARTESIAN_POINT('',(-0.519354515801077,0.75,-1.13462523166105));
#26410=CARTESIAN_POINT('Origin',(0.,0.75,0.));
#26411=CARTESIAN_POINT('',(-0.612662169561028,0.75,-1.08708260743774));
#26412=CARTESIAN_POINT('Origin',(-0.557654483764164,0.75,-1.0944585482776));
#26413=CARTESIAN_POINT('',(-0.690454891028201,0.75,-1.0394111664111));
#26414=CARTESIAN_POINT('Origin',(0.,0.75,0.));
#26415=CARTESIAN_POINT('',(-0.775176467748211,0.75,-0.977857337884348));
#26416=CARTESIAN_POINT('Origin',(-0.721999869202979,0.75,-0.993747566553533));
#26417=CARTESIAN_POINT('',(-0.844553975349804,0.75,-0.918603348636233));
#26418=CARTESIAN_POINT('Origin',(0.,0.75,0.));
#26419=CARTESIAN_POINT('',(-0.918603348636233,0.75,-0.844553975349804));
#26420=CARTESIAN_POINT('Origin',(-0.86856722168183,0.75,-0.86856722168183));
#26421=CARTESIAN_POINT('',(-0.977857337884349,0.75,-0.775176467748211));
#26422=CARTESIAN_POINT('Origin',(0.,0.75,0.));
#26423=CARTESIAN_POINT('',(-1.0394111664111,0.75,-0.690454891028201));
#26424=CARTESIAN_POINT('Origin',(-0.993747566553533,0.75,-0.721999869202979));
#26425=CARTESIAN_POINT('',(-1.08708260743774,0.75,-0.612662169561029));
#26426=CARTESIAN_POINT('Origin',(0.,0.75,0.));
#26427=CARTESIAN_POINT('',(-1.13462523166105,0.75,-0.519354515801077));
#26428=CARTESIAN_POINT('Origin',(-1.0944585482776,0.75,-0.557654483764164));
#26429=CARTESIAN_POINT('',(-1.16954029537568,0.75,-0.435062095450087));
#26430=CARTESIAN_POINT('Origin',(0.,0.75,0.));
#26431=CARTESIAN_POINT('',(-1.20190105810224,0.75,-0.335465908756113));
#26432=CARTESIAN_POINT('Origin',(-1.1682203282434,0.75,-0.379577794185951));
#26433=CARTESIAN_POINT('',(-1.22320001975977,0.75,-0.246749348660852));
#26434=CARTESIAN_POINT('Origin',(0.,0.75,0.));
#26435=CARTESIAN_POINT('',(-1.23958209161204,0.75,-0.143317017690053));
#26436=CARTESIAN_POINT('Origin',(-1.21321664662686,0.75,-0.192154639568406));
#26437=CARTESIAN_POINT('',(-1.24674050008925,0.75,-0.0523608139934482));
#26438=CARTESIAN_POINT('Origin',(0.,0.75,0.));
#26439=CARTESIAN_POINT('',(-1.24674050008925,0.75,0.0523608139934479));
#26440=CARTESIAN_POINT('Origin',(-1.22833954473516,0.75,-1.50428209172603E-16));
#26441=CARTESIAN_POINT('',(-1.23958209161204,0.75,0.143317017690053));
#26442=CARTESIAN_POINT('Origin',(0.,0.75,0.));
#26443=CARTESIAN_POINT('',(-1.22320001975977,0.75,0.246749348660851));
#26444=CARTESIAN_POINT('Origin',(-1.21321664662686,0.75,0.192154639568406));
#26445=CARTESIAN_POINT('',(-1.20190105810224,0.75,0.335465908756113));
#26446=CARTESIAN_POINT('Origin',(0.,0.75,0.));
#26447=CARTESIAN_POINT('',(-1.16954029537568,0.75,0.435062095450087));
#26448=CARTESIAN_POINT('Origin',(-1.1682203282434,0.75,0.379577794185951));
#26449=CARTESIAN_POINT('',(-1.13462523166105,0.75,0.519354515801077));
#26450=CARTESIAN_POINT('Origin',(0.,0.75,0.));
#26451=CARTESIAN_POINT('',(-1.08708260743774,0.75,0.612662169561028));
#26452=CARTESIAN_POINT('Origin',(-1.0944585482776,0.75,0.557654483764164));
#26453=CARTESIAN_POINT('',(-1.0394111664111,0.75,0.690454891028201));
#26454=CARTESIAN_POINT('Origin',(0.,0.75,0.));
#26455=CARTESIAN_POINT('',(-0.977857337884348,0.75,0.775176467748211));
#26456=CARTESIAN_POINT('Origin',(-0.993747566553533,0.75,0.721999869202979));
#26457=CARTESIAN_POINT('',(-0.918603348636233,0.75,0.844553975349804));
#26458=CARTESIAN_POINT('Origin',(0.,0.75,0.));
#26459=CARTESIAN_POINT('',(-0.844553975349804,0.75,0.918603348636233));
#26460=CARTESIAN_POINT('Origin',(-0.86856722168183,0.75,0.86856722168183));
#26461=CARTESIAN_POINT('',(-0.775176467748211,0.75,0.977857337884349));
#26462=CARTESIAN_POINT('Origin',(0.,0.75,0.));
#26463=CARTESIAN_POINT('',(-0.690454891028201,0.75,1.0394111664111));
#26464=CARTESIAN_POINT('Origin',(-0.721999869202979,0.75,0.993747566553533));
#26465=CARTESIAN_POINT('',(-0.612662169561029,0.75,1.08708260743774));
#26466=CARTESIAN_POINT('Origin',(0.,0.75,0.));
#26467=CARTESIAN_POINT('',(-0.519354515801077,0.75,1.13462523166105));
#26468=CARTESIAN_POINT('Origin',(-0.557654483764164,0.75,1.0944585482776));
#26469=CARTESIAN_POINT('',(-0.435062095450087,0.75,1.16954029537568));
#26470=CARTESIAN_POINT('Origin',(0.,0.75,0.));
#26471=CARTESIAN_POINT('',(-0.335465908756113,0.75,1.20190105810224));
#26472=CARTESIAN_POINT('Origin',(-0.379577794185951,0.75,1.1682203282434));
#26473=CARTESIAN_POINT('',(-0.246749348660852,0.75,1.22320001975977));
#26474=CARTESIAN_POINT('Origin',(0.,0.75,0.));
#26475=CARTESIAN_POINT('',(-0.143317017690053,0.75,1.23958209161204));
#26476=CARTESIAN_POINT('Origin',(-0.192154639568406,0.75,1.21321664662686));
#26477=CARTESIAN_POINT('',(-0.0523608139934483,0.75,1.24674050008925));
#26478=CARTESIAN_POINT('Origin',(0.,0.75,0.));
#26479=CARTESIAN_POINT('',(0.0523608139934478,0.75,1.24674050008925));
#26480=CARTESIAN_POINT('Origin',(-2.25642313758905E-16,0.75,1.22833954473516));
#26481=CARTESIAN_POINT('',(0.143317017690053,0.75,1.23958209161204));
#26482=CARTESIAN_POINT('Origin',(0.,0.75,0.));
#26483=CARTESIAN_POINT('',(0.246749348660851,0.75,1.22320001975977));
#26484=CARTESIAN_POINT('Origin',(0.192154639568406,0.75,1.21321664662686));
#26485=CARTESIAN_POINT('',(0.335465908756113,0.75,1.20190105810224));
#26486=CARTESIAN_POINT('Origin',(0.,0.75,0.));
#26487=CARTESIAN_POINT('',(0.435062095450087,0.75,1.16954029537568));
#26488=CARTESIAN_POINT('Origin',(0.379577794185951,0.75,1.1682203282434));
#26489=CARTESIAN_POINT('',(0.519354515801077,0.75,1.13462523166105));
#26490=CARTESIAN_POINT('Origin',(0.,0.75,0.));
#26491=CARTESIAN_POINT('',(0.612662169561028,0.75,1.08708260743774));
#26492=CARTESIAN_POINT('Origin',(0.557654483764164,0.75,1.0944585482776));
#26493=CARTESIAN_POINT('',(0.690454891028201,0.75,1.0394111664111));
#26494=CARTESIAN_POINT('Origin',(0.,0.75,0.));
#26495=CARTESIAN_POINT('',(0.775176467748211,0.75,0.977857337884349));
#26496=CARTESIAN_POINT('Origin',(0.721999869202979,0.75,0.993747566553533));
#26497=CARTESIAN_POINT('',(0.844553975349804,0.75,0.918603348636233));
#26498=CARTESIAN_POINT('Origin',(0.,0.75,0.));
#26499=CARTESIAN_POINT('',(0.918603348636233,0.75,0.844553975349804));
#26500=CARTESIAN_POINT('Origin',(0.86856722168183,0.75,0.86856722168183));
#26501=CARTESIAN_POINT('',(0.977857337884349,0.75,0.775176467748211));
#26502=CARTESIAN_POINT('Origin',(0.,0.75,0.));
#26503=CARTESIAN_POINT('',(1.0394111664111,0.75,0.690454891028201));
#26504=CARTESIAN_POINT('Origin',(0.993747566553533,0.75,0.72199986920298));
#26505=CARTESIAN_POINT('',(1.08708260743774,0.75,0.612662169561029));
#26506=CARTESIAN_POINT('Origin',(0.,0.75,0.));
#26507=CARTESIAN_POINT('',(1.13462523166105,0.75,0.519354515801077));
#26508=CARTESIAN_POINT('Origin',(1.0944585482776,0.75,0.557654483764164));
#26509=CARTESIAN_POINT('',(1.16954029537568,0.75,0.435062095450087));
#26510=CARTESIAN_POINT('Origin',(0.,0.75,0.));
#26511=CARTESIAN_POINT('',(1.20190105810224,0.75,0.335465908756113));
#26512=CARTESIAN_POINT('Origin',(1.1682203282434,0.75,0.379577794185952));
#26513=CARTESIAN_POINT('Origin',(0.,0.75,0.));
#26514=CARTESIAN_POINT('Origin',(0.,0.75,0.));
#26515=CARTESIAN_POINT('',(-1.4,0.85,1.71450551880629E-16));
#26516=CARTESIAN_POINT('Origin',(0.,0.85,0.));
#26517=CARTESIAN_POINT('',(-1.4,0.75,1.71450551880629E-16));
#26518=CARTESIAN_POINT('Origin',(0.,0.85,0.));
#26519=CARTESIAN_POINT('Origin',(1.21321664662686,0.,0.192154639568406));
#26520=CARTESIAN_POINT('',(1.23958209161204,0.,0.14331701769005));
#26521=CARTESIAN_POINT('',(1.22320001975977,0.,0.246749348660855));
#26522=CARTESIAN_POINT('Origin',(0.,0.,0.));
#26523=CARTESIAN_POINT('',(1.20190105810224,0.,0.33546590875611));
#26524=CARTESIAN_POINT('Origin',(1.1682203282434,0.,0.379577794185952));
#26525=CARTESIAN_POINT('',(1.16954029537568,0.,0.43506209545009));
#26526=CARTESIAN_POINT('Origin',(0.,0.,0.));
#26527=CARTESIAN_POINT('',(1.13462523166105,0.,0.519354515801074));
#26528=CARTESIAN_POINT('Origin',(1.0944585482776,0.,0.557654483764164));
#26529=CARTESIAN_POINT('',(1.08708260743774,0.,0.612662169561031));
#26530=CARTESIAN_POINT('Origin',(0.,0.,0.));
#26531=CARTESIAN_POINT('',(1.03941116641111,0.,0.690454891028199));
#26532=CARTESIAN_POINT('Origin',(0.993747566553533,0.,0.72199986920298));
#26533=CARTESIAN_POINT('',(0.977857337884347,0.,0.775176467748214));
#26534=CARTESIAN_POINT('Origin',(0.,0.,0.));
#26535=CARTESIAN_POINT('',(0.918603348636235,0.,0.844553975349802));
#26536=CARTESIAN_POINT('Origin',(0.86856722168183,0.,0.86856722168183));
#26537=CARTESIAN_POINT('',(0.844553975349802,0.,0.918603348636235));
#26538=CARTESIAN_POINT('Origin',(0.,0.,0.));
#26539=CARTESIAN_POINT('',(0.775176467748213,0.,0.977857337884347));
#26540=CARTESIAN_POINT('Origin',(0.721999869202979,0.,0.993747566553533));
#26541=CARTESIAN_POINT('',(0.690454891028198,0.,1.03941116641111));
#26542=CARTESIAN_POINT('Origin',(0.,0.,0.));
#26543=CARTESIAN_POINT('',(0.612662169561031,0.,1.08708260743774));
#26544=CARTESIAN_POINT('Origin',(0.557654483764164,0.,1.0944585482776));
#26545=CARTESIAN_POINT('',(0.519354515801074,0.,1.13462523166105));
#26546=CARTESIAN_POINT('Origin',(0.,0.,0.));
#26547=CARTESIAN_POINT('',(0.43506209545009,0.,1.16954029537568));
#26548=CARTESIAN_POINT('Origin',(0.379577794185951,0.,1.1682203282434));
#26549=CARTESIAN_POINT('',(0.33546590875611,0.,1.20190105810224));
#26550=CARTESIAN_POINT('Origin',(0.,0.,0.));
#26551=CARTESIAN_POINT('',(0.246749348660854,0.,1.22320001975977));
#26552=CARTESIAN_POINT('Origin',(0.192154639568406,0.,1.21321664662686));
#26553=CARTESIAN_POINT('',(0.14331701769005,0.,1.23958209161204));
#26554=CARTESIAN_POINT('Origin',(0.,0.,0.));
#26555=CARTESIAN_POINT('',(0.0523608139934508,0.,1.24674050008925));
#26556=CARTESIAN_POINT('Origin',(-2.25642313758905E-16,0.,1.22833954473516));
#26557=CARTESIAN_POINT('',(-0.0523608139934513,0.,1.24674050008925));
#26558=CARTESIAN_POINT('Origin',(0.,0.,0.));
#26559=CARTESIAN_POINT('',(-0.14331701769005,0.,1.23958209161204));
#26560=CARTESIAN_POINT('Origin',(-0.192154639568406,0.,1.21321664662686));
#26561=CARTESIAN_POINT('',(-0.246749348660855,0.,1.22320001975977));
#26562=CARTESIAN_POINT('Origin',(0.,0.,0.));
#26563=CARTESIAN_POINT('',(-0.33546590875611,0.,1.20190105810224));
#26564=CARTESIAN_POINT('Origin',(-0.379577794185951,0.,1.1682203282434));
#26565=CARTESIAN_POINT('',(-0.43506209545009,0.,1.16954029537568));
#26566=CARTESIAN_POINT('Origin',(0.,0.,0.));
#26567=CARTESIAN_POINT('',(-0.519354515801074,0.,1.13462523166105));
#26568=CARTESIAN_POINT('Origin',(-0.557654483764164,0.,1.0944585482776));
#26569=CARTESIAN_POINT('',(-0.612662169561031,0.,1.08708260743774));
#26570=CARTESIAN_POINT('Origin',(0.,0.,0.));
#26571=CARTESIAN_POINT('',(-0.690454891028199,0.,1.03941116641111));
#26572=CARTESIAN_POINT('Origin',(-0.721999869202979,0.,0.993747566553533));
#26573=CARTESIAN_POINT('',(-0.775176467748213,0.,0.977857337884347));
#26574=CARTESIAN_POINT('Origin',(0.,0.,0.));
#26575=CARTESIAN_POINT('',(-0.844553975349802,0.,0.918603348636235));
#26576=CARTESIAN_POINT('Origin',(-0.86856722168183,0.,0.86856722168183));
#26577=CARTESIAN_POINT('',(-0.918603348636235,0.,0.844553975349802));
#26578=CARTESIAN_POINT('Origin',(0.,0.,0.));
#26579=CARTESIAN_POINT('',(-0.977857337884347,0.,0.775176467748213));
#26580=CARTESIAN_POINT('Origin',(-0.993747566553533,0.,0.721999869202979));
#26581=CARTESIAN_POINT('',(-1.03941116641111,0.,0.690454891028198));
#26582=CARTESIAN_POINT('Origin',(0.,0.,0.));
#26583=CARTESIAN_POINT('',(-1.08708260743774,0.,0.612662169561031));
#26584=CARTESIAN_POINT('Origin',(-1.0944585482776,0.,0.557654483764164));
#26585=CARTESIAN_POINT('',(-1.13462523166105,0.,0.519354515801074));
#26586=CARTESIAN_POINT('Origin',(0.,0.,0.));
#26587=CARTESIAN_POINT('',(-1.16954029537568,0.,0.43506209545009));
#26588=CARTESIAN_POINT('Origin',(-1.1682203282434,0.,0.379577794185951));
#26589=CARTESIAN_POINT('',(-1.20190105810224,0.,0.33546590875611));
#26590=CARTESIAN_POINT('Origin',(0.,0.,0.));
#26591=CARTESIAN_POINT('',(-1.22320001975977,0.,0.246749348660854));
#26592=CARTESIAN_POINT('Origin',(-1.21321664662686,0.,0.192154639568406));
#26593=CARTESIAN_POINT('',(-1.23958209161204,0.,0.14331701769005));
#26594=CARTESIAN_POINT('Origin',(0.,0.,0.));
#26595=CARTESIAN_POINT('',(-1.24674050008925,0.,0.0523608139934509));
#26596=CARTESIAN_POINT('Origin',(-1.22833954473516,0.,-1.50428209172603E-16));
#26597=CARTESIAN_POINT('',(-1.24674050008925,0.,-0.0523608139934512));
#26598=CARTESIAN_POINT('Origin',(0.,0.,0.));
#26599=CARTESIAN_POINT('',(-1.23958209161204,0.,-0.14331701769005));
#26600=CARTESIAN_POINT('Origin',(-1.21321664662686,0.,-0.192154639568406));
#26601=CARTESIAN_POINT('',(-1.22320001975977,0.,-0.246749348660855));
#26602=CARTESIAN_POINT('Origin',(0.,0.,0.));
#26603=CARTESIAN_POINT('',(-1.20190105810224,0.,-0.33546590875611));
#26604=CARTESIAN_POINT('Origin',(-1.1682203282434,0.,-0.379577794185951));
#26605=CARTESIAN_POINT('',(-1.16954029537568,0.,-0.43506209545009));
#26606=CARTESIAN_POINT('Origin',(0.,0.,0.));
#26607=CARTESIAN_POINT('',(-1.13462523166105,0.,-0.519354515801074));
#26608=CARTESIAN_POINT('Origin',(-1.0944585482776,0.,-0.557654483764164));
#26609=CARTESIAN_POINT('',(-1.08708260743774,0.,-0.612662169561031));
#26610=CARTESIAN_POINT('Origin',(0.,0.,0.));
#26611=CARTESIAN_POINT('',(-1.03941116641111,0.,-0.690454891028199));
#26612=CARTESIAN_POINT('Origin',(-0.993747566553533,0.,-0.721999869202979));
#26613=CARTESIAN_POINT('',(-0.977857337884347,0.,-0.775176467748213));
#26614=CARTESIAN_POINT('Origin',(0.,0.,0.));
#26615=CARTESIAN_POINT('',(-0.918603348636235,0.,-0.844553975349802));
#26616=CARTESIAN_POINT('Origin',(-0.86856722168183,0.,-0.86856722168183));
#26617=CARTESIAN_POINT('',(-0.844553975349802,0.,-0.918603348636235));
#26618=CARTESIAN_POINT('Origin',(0.,0.,0.));
#26619=CARTESIAN_POINT('',(-0.775176467748213,0.,-0.977857337884347));
#26620=CARTESIAN_POINT('Origin',(-0.721999869202979,0.,-0.993747566553533));
#26621=CARTESIAN_POINT('',(-0.690454891028198,0.,-1.03941116641111));
#26622=CARTESIAN_POINT('Origin',(0.,0.,0.));
#26623=CARTESIAN_POINT('',(-0.612662169561031,0.,-1.08708260743774));
#26624=CARTESIAN_POINT('Origin',(-0.557654483764164,0.,-1.0944585482776));
#26625=CARTESIAN_POINT('',(-0.519354515801074,0.,-1.13462523166105));
#26626=CARTESIAN_POINT('Origin',(0.,0.,0.));
#26627=CARTESIAN_POINT('',(-0.43506209545009,0.,-1.16954029537568));
#26628=CARTESIAN_POINT('Origin',(-0.379577794185951,0.,-1.1682203282434));
#26629=CARTESIAN_POINT('',(-0.33546590875611,0.,-1.20190105810224));
#26630=CARTESIAN_POINT('Origin',(0.,0.,0.));
#26631=CARTESIAN_POINT('',(-0.246749348660854,0.,-1.22320001975977));
#26632=CARTESIAN_POINT('Origin',(-0.192154639568406,0.,-1.21321664662686));
#26633=CARTESIAN_POINT('',(-0.14331701769005,0.,-1.23958209161204));
#26634=CARTESIAN_POINT('Origin',(0.,0.,0.));
#26635=CARTESIAN_POINT('',(-0.052360813993451,0.,-1.24674050008925));
#26636=CARTESIAN_POINT('Origin',(7.52141045863017E-17,0.,-1.22833954473516));
#26637=CARTESIAN_POINT('',(0.0523608139934511,0.,-1.24674050008925));
#26638=CARTESIAN_POINT('Origin',(0.,0.,0.));
#26639=CARTESIAN_POINT('',(0.14331701769005,0.,-1.23958209161204));
#26640=CARTESIAN_POINT('Origin',(0.192154639568406,0.,-1.21321664662686));
#26641=CARTESIAN_POINT('',(0.246749348660855,0.,-1.22320001975977));
#26642=CARTESIAN_POINT('Origin',(0.,0.,0.));
#26643=CARTESIAN_POINT('',(0.33546590875611,0.,-1.20190105810224));
#26644=CARTESIAN_POINT('Origin',(0.379577794185951,0.,-1.1682203282434));
#26645=CARTESIAN_POINT('',(0.43506209545009,0.,-1.16954029537568));
#26646=CARTESIAN_POINT('Origin',(0.,0.,0.));
#26647=CARTESIAN_POINT('',(0.519354515801074,0.,-1.13462523166105));
#26648=CARTESIAN_POINT('Origin',(0.557654483764164,0.,-1.0944585482776));
#26649=CARTESIAN_POINT('',(0.612662169561031,0.,-1.08708260743774));
#26650=CARTESIAN_POINT('Origin',(0.,0.,0.));
#26651=CARTESIAN_POINT('',(0.690454891028198,0.,-1.03941116641111));
#26652=CARTESIAN_POINT('Origin',(0.721999869202979,0.,-0.993747566553533));
#26653=CARTESIAN_POINT('',(0.775176467748213,0.,-0.977857337884347));
#26654=CARTESIAN_POINT('Origin',(0.,0.,0.));
#26655=CARTESIAN_POINT('',(0.844553975349802,0.,-0.918603348636235));
#26656=CARTESIAN_POINT('Origin',(0.86856722168183,0.,-0.86856722168183));
#26657=CARTESIAN_POINT('',(0.918603348636235,0.,-0.844553975349802));
#26658=CARTESIAN_POINT('Origin',(0.,0.,0.));
#26659=CARTESIAN_POINT('',(0.977857337884347,0.,-0.775176467748213));
#26660=CARTESIAN_POINT('Origin',(0.993747566553533,0.,-0.721999869202979));
#26661=CARTESIAN_POINT('',(1.03941116641111,0.,-0.690454891028198));
#26662=CARTESIAN_POINT('Origin',(0.,0.,0.));
#26663=CARTESIAN_POINT('',(1.08708260743774,0.,-0.612662169561031));
#26664=CARTESIAN_POINT('Origin',(1.0944585482776,0.,-0.557654483764164));
#26665=CARTESIAN_POINT('',(1.13462523166105,0.,-0.519354515801074));
#26666=CARTESIAN_POINT('Origin',(0.,0.,0.));
#26667=CARTESIAN_POINT('',(1.16954029537568,0.,-0.43506209545009));
#26668=CARTESIAN_POINT('Origin',(1.1682203282434,0.,-0.379577794185951));
#26669=CARTESIAN_POINT('',(1.20190105810224,0.,-0.33546590875611));
#26670=CARTESIAN_POINT('Origin',(0.,0.,0.));
#26671=CARTESIAN_POINT('',(1.22320001975977,0.,-0.246749348660855));
#26672=CARTESIAN_POINT('Origin',(1.21321664662686,0.,-0.192154639568406));
#26673=CARTESIAN_POINT('',(1.23958209161204,0.,-0.14331701769005));
#26674=CARTESIAN_POINT('Origin',(0.,0.,0.));
#26675=CARTESIAN_POINT('',(1.24674050008925,0.,0.052360813993451));
#26676=CARTESIAN_POINT('Origin',(1.22833954473516,0.,0.));
#26677=CARTESIAN_POINT('',(1.24674050008925,0.,-0.052360813993451));
#26678=CARTESIAN_POINT('Origin',(0.,0.,0.));
#26989=UNCERTAINTY_MEASURE_WITH_UNIT(LENGTH_MEASURE(0.001),#27070,
'DISTANCE_ACCURACY_VALUE',
'Maximum model space distance between geometric entities at asserted c
onnectivities');
#26992=UNCERTAINTY_MEASURE_WITH_UNIT(LENGTH_MEASURE(0.001),#27070,
'DISTANCE_ACCURACY_VALUE',
'Maximum model space distance between geometric entities at asserted c
onnectivities');
#27066=(
GEOMETRIC_REPRESENTATION_CONTEXT(3)
GLOBAL_UNCERTAINTY_ASSIGNED_CONTEXT((#26989))
GLOBAL_UNIT_ASSIGNED_CONTEXT((#27070,#27072,#27073))
REPRESENTATION_CONTEXT('','3D')
);
#27069=(
GEOMETRIC_REPRESENTATION_CONTEXT(3)
GLOBAL_UNCERTAINTY_ASSIGNED_CONTEXT((#26992))
GLOBAL_UNIT_ASSIGNED_CONTEXT((#27070,#27072,#27073))
REPRESENTATION_CONTEXT('','3D')
);
#27070=(
LENGTH_UNIT()
NAMED_UNIT(*)
SI_UNIT(.CENTI.,.METRE.)
);
#27072=(
NAMED_UNIT(*)
PLANE_ANGLE_UNIT()
SI_UNIT($,.RADIAN.)
);
#27073=(
NAMED_UNIT(*)
SI_UNIT($,.STERADIAN.)
SOLID_ANGLE_UNIT()
);
#27147=SHAPE_DEFINITION_REPRESENTATION(#27235,#27424);
#27235=PRODUCT_DEFINITION_SHAPE('',$,#27501);
#27424=SHAPE_REPRESENTATION('',(#16016),#27066);
#27427=PRODUCT_DEFINITION_CONTEXT('part definition',#27657,'design');
#27501=PRODUCT_DEFINITION(
'Timing Pulley - 2 mm Pitch, 40 Teeth, 12 mm Bore',
'Timing Pulley - 2 mm Pitch, 40 Teeth, 12 mm Bore',#27577,#27427);
#27577=PRODUCT_DEFINITION_FORMATION('',$,#27732);
#27657=APPLICATION_CONTEXT(
'Core Data for Automotive Mechanical Design Process');
#27658=PRODUCT_CONTEXT('part definition',#27657,'mechanical');
#27732=PRODUCT('Timing Pulley - 2 mm Pitch, 40 Teeth, 12 mm Bore',
'Timing Pulley - 2 mm Pitch, 40 Teeth, 12 mm Bore',
'Timing Pulley - 2 mm Pitch, 40 Teeth, 12 mm Bore',(#27658));
#27784=COLOUR_RGB('Sky Blue',0.24,0.69,0.87);
#27785=FILL_AREA_STYLE_COLOUR('',#27784);
#27786=FILL_AREA_STYLE('',(#27785));
#27787=SURFACE_STYLE_FILL_AREA(#27786);
#27788=SURFACE_SIDE_STYLE('',(#27787));
#27789=SURFACE_STYLE_USAGE(.BOTH.,#27788);
#27790=PRESENTATION_STYLE_ASSIGNMENT((#27789));
ENDSEC;
END-ISO-10303-21;
